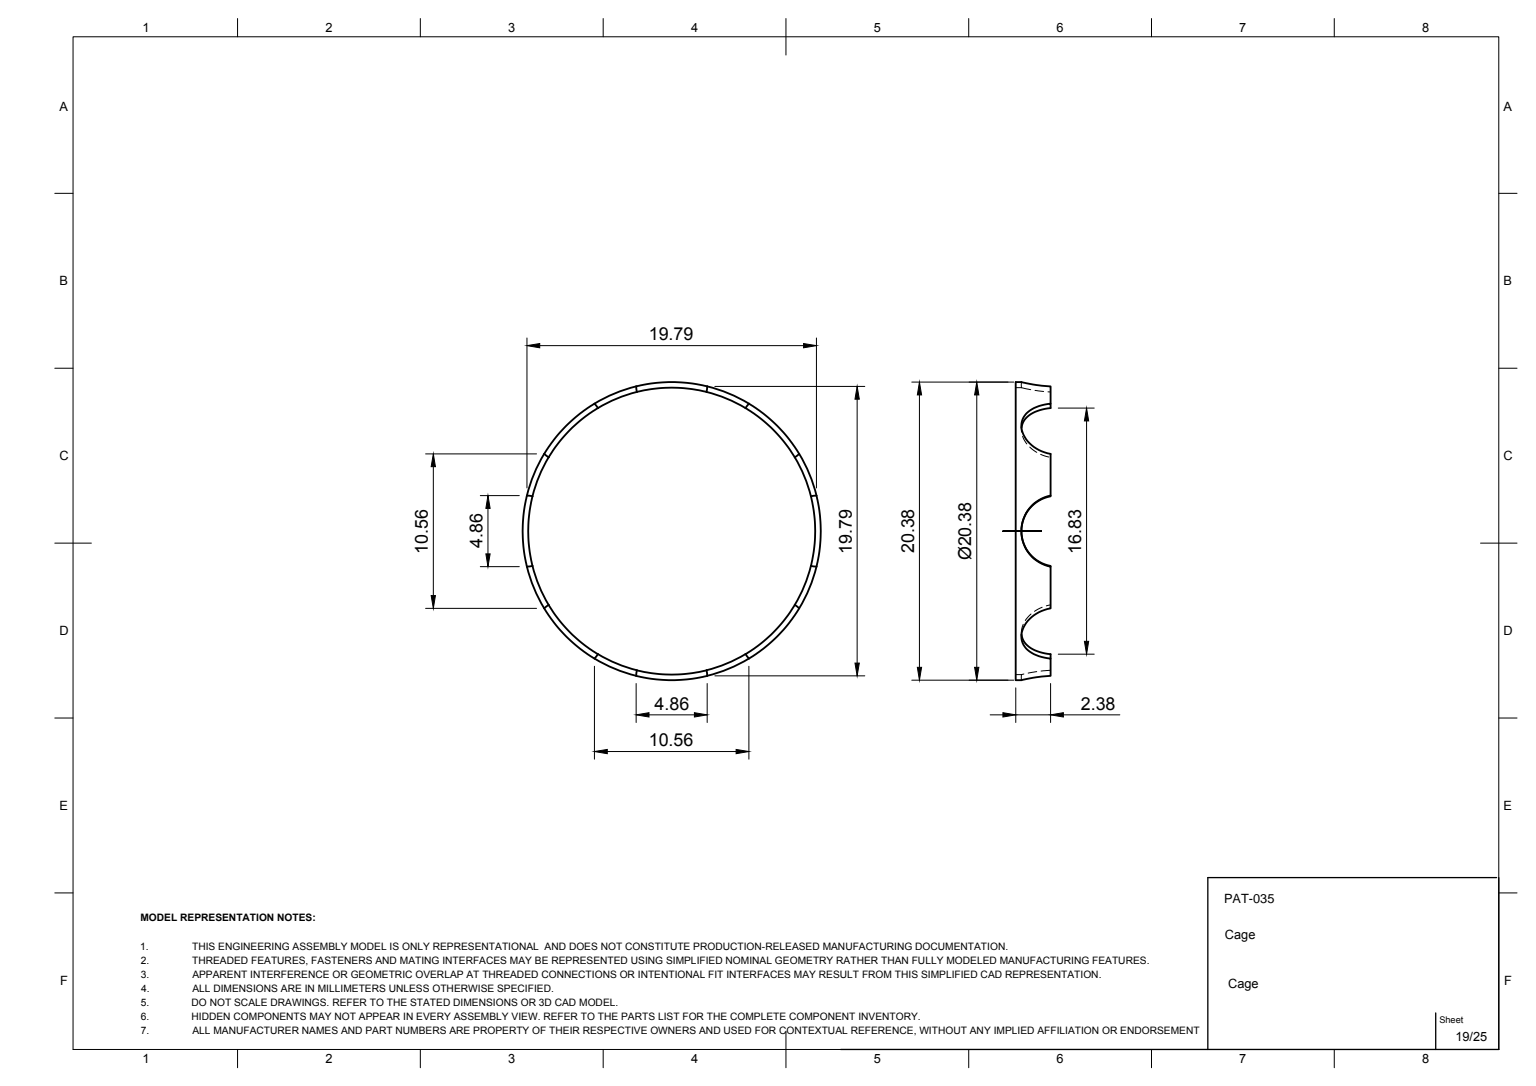
ISO-10303-21;
HEADER;
/* Generated by software containing ST-Developer
 * from STEP Tools, Inc. (www.steptools.com) 
 */

FILE_DESCRIPTION(
/* description */ ('Five-roller gravity conveyor'),
/* implementation_level */ '2;1');

FILE_NAME(
/* name */ 'Cage.step',
/* time_stamp */ '2026-10-29T15:36:43-07:00',
/* author */ (''),
/* organization */ (''),
/* preprocessor_version */ 'ST-DEVELOPER v20.2',
/* originating_system */ 'Autodesk Translation Framework v15.17.0.0',
/* authorisation */ '');

FILE_SCHEMA (('AUTOMOTIVE_DESIGN { 1 0 10303 214 3 1 1 }'));
ENDSEC;

DATA;
#10=MECHANICAL_DESIGN_GEOMETRIC_PRESENTATION_REPRESENTATION('',(#328),#7806);
#223=B_SPLINE_CURVE_WITH_KNOTS('',3,(#7017,#7018,#7019,#7020,#7021,#7022,
#7023,#7024,#7025,#7026,#7027,#7028,#7029,#7030,#7031,#7032,#7033,#7034,
#7035,#7036,#7037,#7038),.UNSPECIFIED.,.F.,.F.,(4,2,2,2,2,2,2,2,2,2,4),
(0.0473477652366656,0.126350602536658,0.189525903804987,0.252701205073317,
0.313298422430275,0.373895639787233,0.434492857144191,0.495090074501149,
0.558265375769478,0.621440677037807,0.7004435143378),.UNSPECIFIED.);
#224=B_SPLINE_CURVE_WITH_KNOTS('',3,(#7042,#7043,#7044,#7045,#7046,#7047,
#7048,#7049,#7050,#7051,#7052,#7053,#7054,#7055,#7056,#7057,#7058,#7059,
#7060,#7061,#7062,#7063),.UNSPECIFIED.,.F.,.F.,(4,2,2,2,2,2,2,2,2,2,4),
(0.0464897534940957,0.0852567806515119,0.170513561303024,0.246687263103517,
0.308657850341199,0.370628437578881,0.432599024816563,0.494569612054245,
0.570743313854739,0.656000094506251,0.694767121663666),.UNSPECIFIED.);
#225=B_SPLINE_CURVE_WITH_KNOTS('',3,(#7069,#7070,#7071,#7072,#7073,#7074,
#7075,#7076,#7077,#7078,#7079,#7080,#7081,#7082,#7083,#7084,#7085,#7086,
#7087,#7088,#7089,#7090),.UNSPECIFIED.,.F.,.F.,(4,2,2,2,2,2,2,2,2,2,4),
(0.0464897534940957,0.0852567806515118,0.170513561303024,0.246687263103517,
0.308657850341199,0.370628437578881,0.432599024816563,0.494569612054245,
0.570743313854738,0.65600009450625,0.694767121663666),.UNSPECIFIED.);
#226=B_SPLINE_CURVE_WITH_KNOTS('',3,(#7094,#7095,#7096,#7097,#7098,#7099,
#7100,#7101,#7102,#7103,#7104,#7105,#7106,#7107,#7108,#7109,#7110,#7111,
#7112,#7113,#7114,#7115),.UNSPECIFIED.,.F.,.F.,(4,2,2,2,2,2,2,2,2,2,4),
(0.0464897534940957,0.0852567806515119,0.170513561303024,0.246687263103517,
0.308657850341199,0.370628437578881,0.432599024816563,0.494569612054245,
0.570743313854739,0.656000094506251,0.694767121663666),.UNSPECIFIED.);
#227=B_SPLINE_CURVE_WITH_KNOTS('',3,(#7119,#7120,#7121,#7122,#7123,#7124,
#7125,#7126,#7127,#7128,#7129,#7130),.UNSPECIFIED.,.F.,.F.,(4,2,2,2,2,4),
(0.0464897534940957,0.0852567806515119,0.170513561303024,0.246687263103517,
0.308657850341199,0.370628437578881),.UNSPECIFIED.);
#228=B_SPLINE_CURVE_WITH_KNOTS('',3,(#7135,#7136,#7137,#7138,#7139,#7140,
#7141,#7142,#7143,#7144,#7145,#7146),.UNSPECIFIED.,.F.,.F.,(4,2,2,2,2,4),
(0.370628437578881,0.432599024816563,0.494569612054245,0.570743313854738,
0.65600009450625,0.694767121663666),.UNSPECIFIED.);
#229=B_SPLINE_CURVE_WITH_KNOTS('',3,(#7150,#7151,#7152,#7153,#7154,#7155,
#7156,#7157,#7158,#7159,#7160,#7161,#7162,#7163,#7164,#7165,#7166,#7167,
#7168,#7169,#7170,#7171),.UNSPECIFIED.,.F.,.F.,(4,2,2,2,2,2,2,2,2,2,4),
(0.0464897534940957,0.0852567806515121,0.170513561303024,0.246687263103518,
0.308657850341199,0.370628437578881,0.432599024816563,0.494569612054245,
0.570743313854738,0.65600009450625,0.694767121663666),.UNSPECIFIED.);
#230=B_SPLINE_CURVE_WITH_KNOTS('',3,(#7175,#7176,#7177,#7178,#7179,#7180,
#7181,#7182,#7183,#7184,#7185,#7186,#7187,#7188,#7189,#7190,#7191,#7192,
#7193,#7194,#7195,#7196),.UNSPECIFIED.,.F.,.F.,(4,2,2,2,2,2,2,2,2,2,4),
(0.0464897534940957,0.0852567806515119,0.170513561303024,0.246687263103517,
0.308657850341199,0.370628437578881,0.432599024816563,0.494569612054245,
0.570743313854738,0.65600009450625,0.694767121663667),.UNSPECIFIED.);
#231=B_SPLINE_CURVE_WITH_KNOTS('',3,(#7200,#7201,#7202,#7203,#7204,#7205,
#7206,#7207,#7208,#7209,#7210,#7211,#7212,#7213,#7214,#7215,#7216,#7217,
#7218,#7219,#7220,#7221),.UNSPECIFIED.,.F.,.F.,(4,2,2,2,2,2,2,2,2,2,4),
(0.0464897534940957,0.0852567806515119,0.170513561303024,0.246687263103517,
0.308657850341199,0.370628437578881,0.432599024816563,0.494569612054245,
0.570743313854738,0.65600009450625,0.694767121663666),.UNSPECIFIED.);
#232=B_SPLINE_CURVE_WITH_KNOTS('',3,(#7225,#7226,#7227,#7228,#7229,#7230,
#7231,#7232,#7233,#7234,#7235,#7236,#7237,#7238,#7239,#7240,#7241,#7242,
#7243,#7244,#7245,#7246),.UNSPECIFIED.,.F.,.F.,(4,2,2,2,2,2,2,2,2,2,4),
(0.0464897534940957,0.0852567806515119,0.170513561303024,0.246687263103517,
0.308657850341199,0.370628437578881,0.432599024816563,0.494569612054245,
0.570743313854739,0.656000094506251,0.694767121663667),.UNSPECIFIED.);
#233=B_SPLINE_CURVE_WITH_KNOTS('',3,(#7254,#7255,#7256,#7257,#7258,#7259,
#7260,#7261,#7262,#7263,#7264,#7265,#7266,#7267,#7268,#7269,#7270,#7271,
#7272,#7273,#7274,#7275),.UNSPECIFIED.,.F.,.F.,(4,2,2,2,2,2,2,2,2,2,4),
(0.0473477652366656,0.126350602536658,0.189525903804987,0.252701205073316,
0.313298422430274,0.373895639787232,0.434492857144191,0.495090074501149,
0.558265375769478,0.621440677037807,0.7004435143378),.UNSPECIFIED.);
#234=B_SPLINE_CURVE_WITH_KNOTS('',3,(#7283,#7284,#7285,#7286,#7287,#7288,
#7289,#7290,#7291,#7292,#7293,#7294,#7295,#7296,#7297,#7298,#7299,#7300,
#7301,#7302,#7303,#7304),.UNSPECIFIED.,.F.,.F.,(4,2,2,2,2,2,2,2,2,2,4),
(0.0473477652366656,0.126350602536658,0.189525903804987,0.252701205073317,
0.313298422430275,0.373895639787233,0.434492857144191,0.495090074501149,
0.558265375769478,0.621440677037807,0.7004435143378),.UNSPECIFIED.);
#235=B_SPLINE_CURVE_WITH_KNOTS('',3,(#7313,#7314,#7315,#7316,#7317,#7318,
#7319,#7320,#7321,#7322,#7323,#7324),.UNSPECIFIED.,.F.,.F.,(4,2,2,2,2,4),
(0.0473477652366656,0.126350602536658,0.189525903804987,0.252701205073316,
0.313298422430275,0.373895639787233),.UNSPECIFIED.);
#236=B_SPLINE_CURVE_WITH_KNOTS('',3,(#7326,#7327,#7328,#7329,#7330,#7331,
#7332,#7333,#7334,#7335,#7336,#7337),.UNSPECIFIED.,.F.,.F.,(4,2,2,2,2,4),
(0.373895639787233,0.434492857144191,0.495090074501149,0.558265375769478,
0.621440677037807,0.7004435143378),.UNSPECIFIED.);
#237=B_SPLINE_CURVE_WITH_KNOTS('',3,(#7344,#7345,#7346,#7347,#7348,#7349,
#7350,#7351,#7352,#7353,#7354,#7355,#7356,#7357,#7358,#7359,#7360,#7361,
#7362,#7363,#7364,#7365),.UNSPECIFIED.,.F.,.F.,(4,2,2,2,2,2,2,2,2,2,4),
(0.0473477652366656,0.126350602536658,0.189525903804987,0.252701205073316,
0.313298422430275,0.373895639787233,0.434492857144191,0.495090074501149,
0.558265375769478,0.621440677037807,0.7004435143378),.UNSPECIFIED.);
#238=B_SPLINE_CURVE_WITH_KNOTS('',3,(#7373,#7374,#7375,#7376,#7377,#7378,
#7379,#7380,#7381,#7382,#7383,#7384,#7385,#7386,#7387,#7388,#7389,#7390,
#7391,#7392,#7393,#7394),.UNSPECIFIED.,.F.,.F.,(4,2,2,2,2,2,2,2,2,2,4),
(0.0473477652366656,0.126350602536658,0.189525903804987,0.252701205073317,
0.313298422430275,0.373895639787233,0.434492857144191,0.495090074501149,
0.558265375769478,0.621440677037807,0.7004435143378),.UNSPECIFIED.);
#239=B_SPLINE_CURVE_WITH_KNOTS('',3,(#7402,#7403,#7404,#7405,#7406,#7407,
#7408,#7409,#7410,#7411,#7412,#7413,#7414,#7415,#7416,#7417,#7418,#7419,
#7420,#7421,#7422,#7423),.UNSPECIFIED.,.F.,.F.,(4,2,2,2,2,2,2,2,2,2,4),
(0.0473477652366656,0.126350602536658,0.189525903804987,0.252701205073316,
0.313298422430275,0.373895639787233,0.434492857144191,0.495090074501149,
0.558265375769478,0.621440677037807,0.7004435143378),.UNSPECIFIED.);
#240=B_SPLINE_CURVE_WITH_KNOTS('',3,(#7432,#7433,#7434,#7435,#7436,#7437,
#7438,#7439,#7440,#7441,#7442,#7443,#7444,#7445,#7446,#7447,#7448,#7449,
#7450,#7451,#7452,#7453),.UNSPECIFIED.,.F.,.F.,(4,2,2,2,2,2,2,2,2,2,4),
(0.0473477652366656,0.126350602536658,0.189525903804987,0.252701205073317,
0.313298422430275,0.373895639787233,0.434492857144191,0.495090074501149,
0.558265375769478,0.621440677037807,0.7004435143378),.UNSPECIFIED.);
#249=SPHERICAL_SURFACE('',#4677,0.247676);
#250=SPHERICAL_SURFACE('',#4693,0.247676);
#251=SPHERICAL_SURFACE('',#4698,0.247676);
#252=SPHERICAL_SURFACE('',#4703,0.247676);
#253=SPHERICAL_SURFACE('',#4708,0.247676);
#254=SPHERICAL_SURFACE('',#4713,0.247676);
#255=SPHERICAL_SURFACE('',#4718,0.247676);
#256=SPHERICAL_SURFACE('',#4726,0.247676);
#285=SHAPE_REPRESENTATION_RELATIONSHIP('SRR','None',#7923,#303);
#303=ADVANCED_BREP_SHAPE_REPRESENTATION('',(#353),#7796);
#328=STYLED_ITEM('',(#8091),#353);
#353=MANIFOLD_SOLID_BREP('Continuous crown cage',#4216);
#386=FACE_BOUND('',#1080,.T.);
#502=CIRCLE('',#4678,0.243053047864041);
#503=CIRCLE('',#4679,0.243053047864041);
#504=CIRCLE('',#4681,1.019052);
#505=CIRCLE('',#4682,1.019052);
#506=CIRCLE('',#4683,1.019052);
#507=CIRCLE('',#4684,1.019052);
#508=CIRCLE('',#4685,1.019052);
#509=CIRCLE('',#4686,1.019052);
#510=CIRCLE('',#4687,1.019052);
#511=CIRCLE('',#4688,1.019052);
#512=CIRCLE('',#4689,1.019052);
#513=CIRCLE('',#4691,0.980948);
#514=CIRCLE('',#4692,0.243053047864041);
#515=CIRCLE('',#4694,0.243053047864041);
#516=CIRCLE('',#4696,0.980948);
#517=CIRCLE('',#4697,0.243053047864041);
#518=CIRCLE('',#4699,0.243053047864041);
#519=CIRCLE('',#4701,0.980948);
#520=CIRCLE('',#4702,0.243053047864041);
#521=CIRCLE('',#4704,0.243053047864041);
#522=CIRCLE('',#4706,0.980948);
#523=CIRCLE('',#4707,0.243053047864041);
#524=CIRCLE('',#4709,0.243053047864041);
#525=CIRCLE('',#4711,0.980948);
#526=CIRCLE('',#4712,0.243053047864041);
#527=CIRCLE('',#4714,0.243053047864041);
#528=CIRCLE('',#4716,0.980948);
#529=CIRCLE('',#4717,0.243053047864041);
#530=CIRCLE('',#4719,0.243053047864041);
#531=CIRCLE('',#4721,0.980948);
#532=CIRCLE('',#4722,0.980948);
#533=CIRCLE('',#4723,0.980948);
#534=CIRCLE('',#4725,0.243053047864041);
#535=CIRCLE('',#4727,0.243053047864041);
#623=CYLINDRICAL_SURFACE('',#4680,1.019052);
#624=CYLINDRICAL_SURFACE('',#4720,0.980948);
#806=FACE_OUTER_BOUND('',#1062,.T.);
#807=FACE_OUTER_BOUND('',#1063,.T.);
#808=FACE_OUTER_BOUND('',#1064,.T.);
#809=FACE_OUTER_BOUND('',#1065,.T.);
#810=FACE_OUTER_BOUND('',#1066,.T.);
#811=FACE_OUTER_BOUND('',#1067,.T.);
#812=FACE_OUTER_BOUND('',#1068,.T.);
#813=FACE_OUTER_BOUND('',#1069,.T.);
#814=FACE_OUTER_BOUND('',#1070,.T.);
#815=FACE_OUTER_BOUND('',#1071,.T.);
#816=FACE_OUTER_BOUND('',#1072,.T.);
#817=FACE_OUTER_BOUND('',#1073,.T.);
#818=FACE_OUTER_BOUND('',#1074,.T.);
#819=FACE_OUTER_BOUND('',#1075,.T.);
#820=FACE_OUTER_BOUND('',#1076,.T.);
#821=FACE_OUTER_BOUND('',#1077,.T.);
#822=FACE_OUTER_BOUND('',#1078,.T.);
#823=FACE_OUTER_BOUND('',#1079,.T.);
#824=FACE_OUTER_BOUND('',#1081,.T.);
#1062=EDGE_LOOP('',(#3500,#3501,#3502,#3503));
#1063=EDGE_LOOP('',(#3504,#3505,#3506,#3507,#3508,#3509,#3510,#3511,#3512,
#3513,#3514,#3515,#3516,#3517,#3518,#3519,#3520,#3521,#3522,#3523));
#1064=EDGE_LOOP('',(#3524,#3525,#3526,#3527));
#1065=EDGE_LOOP('',(#3528,#3529,#3530,#3531));
#1066=EDGE_LOOP('',(#3532,#3533,#3534,#3535));
#1067=EDGE_LOOP('',(#3536,#3537,#3538,#3539));
#1068=EDGE_LOOP('',(#3540,#3541,#3542,#3543));
#1069=EDGE_LOOP('',(#3544,#3545,#3546,#3547,#3548,#3549));
#1070=EDGE_LOOP('',(#3550,#3551,#3552,#3553));
#1071=EDGE_LOOP('',(#3554,#3555,#3556,#3557));
#1072=EDGE_LOOP('',(#3558,#3559,#3560,#3561));
#1073=EDGE_LOOP('',(#3562,#3563,#3564,#3565));
#1074=EDGE_LOOP('',(#3566,#3567,#3568,#3569));
#1075=EDGE_LOOP('',(#3570,#3571,#3572,#3573));
#1076=EDGE_LOOP('',(#3574,#3575,#3576,#3577,#3578,#3579,#3580,#3581,#3582,
#3583,#3584,#3585,#3586,#3587,#3588,#3589,#3590,#3591,#3592,#3593));
#1077=EDGE_LOOP('',(#3594,#3595,#3596,#3597));
#1078=EDGE_LOOP('',(#3598,#3599,#3600,#3601));
#1079=EDGE_LOOP('',(#3602));
#1080=EDGE_LOOP('',(#3603));
#1081=EDGE_LOOP('',(#3604,#3605,#3606,#3607));
#1465=LINE('',#7132,#1806);
#1466=LINE('',#7428,#1807);
#1806=VECTOR('',#5715,1.019052);
#1807=VECTOR('',#5792,0.980948);
#2114=VERTEX_POINT('',#7015);
#2115=VERTEX_POINT('',#7016);
#2116=VERTEX_POINT('',#7039);
#2117=VERTEX_POINT('',#7041);
#2118=VERTEX_POINT('',#7066);
#2119=VERTEX_POINT('',#7068);
#2120=VERTEX_POINT('',#7091);
#2121=VERTEX_POINT('',#7093);
#2122=VERTEX_POINT('',#7116);
#2123=VERTEX_POINT('',#7118);
#2124=VERTEX_POINT('',#7131);
#2125=VERTEX_POINT('',#7134);
#2126=VERTEX_POINT('',#7147);
#2127=VERTEX_POINT('',#7149);
#2128=VERTEX_POINT('',#7172);
#2129=VERTEX_POINT('',#7174);
#2130=VERTEX_POINT('',#7197);
#2131=VERTEX_POINT('',#7199);
#2132=VERTEX_POINT('',#7222);
#2133=VERTEX_POINT('',#7224);
#2134=VERTEX_POINT('',#7249);
#2135=VERTEX_POINT('',#7253);
#2136=VERTEX_POINT('',#7278);
#2137=VERTEX_POINT('',#7282);
#2138=VERTEX_POINT('',#7307);
#2139=VERTEX_POINT('',#7311);
#2140=VERTEX_POINT('',#7312);
#2141=VERTEX_POINT('',#7339);
#2142=VERTEX_POINT('',#7343);
#2143=VERTEX_POINT('',#7368);
#2144=VERTEX_POINT('',#7372);
#2145=VERTEX_POINT('',#7397);
#2146=VERTEX_POINT('',#7401);
#2147=VERTEX_POINT('',#7426);
#2148=VERTEX_POINT('',#7429);
#2149=VERTEX_POINT('',#7431);
#2593=EDGE_CURVE('',#2114,#2115,#223,.T.);
#2594=EDGE_CURVE('',#2116,#2114,#502,.T.);
#2595=EDGE_CURVE('',#2117,#2116,#224,.T.);
#2596=EDGE_CURVE('',#2115,#2117,#503,.T.);
#2597=EDGE_CURVE('',#2118,#2116,#504,.T.);
#2598=EDGE_CURVE('',#2118,#2119,#225,.T.);
#2599=EDGE_CURVE('',#2120,#2119,#505,.T.);
#2600=EDGE_CURVE('',#2120,#2121,#226,.T.);
#2601=EDGE_CURVE('',#2122,#2121,#506,.T.);
#2602=EDGE_CURVE('',#2122,#2123,#227,.T.);
#2603=EDGE_CURVE('',#2123,#2124,#1465,.T.);
#2604=EDGE_CURVE('',#2124,#2124,#507,.T.);
#2605=EDGE_CURVE('',#2123,#2125,#228,.T.);
#2606=EDGE_CURVE('',#2126,#2125,#508,.T.);
#2607=EDGE_CURVE('',#2126,#2127,#229,.T.);
#2608=EDGE_CURVE('',#2128,#2127,#509,.T.);
#2609=EDGE_CURVE('',#2128,#2129,#230,.T.);
#2610=EDGE_CURVE('',#2130,#2129,#510,.T.);
#2611=EDGE_CURVE('',#2130,#2131,#231,.T.);
#2612=EDGE_CURVE('',#2132,#2131,#511,.T.);
#2613=EDGE_CURVE('',#2132,#2133,#232,.T.);
#2614=EDGE_CURVE('',#2117,#2133,#512,.T.);
#2615=EDGE_CURVE('',#2114,#2134,#513,.T.);
#2616=EDGE_CURVE('',#2134,#2118,#514,.T.);
#2617=EDGE_CURVE('',#2135,#2134,#233,.T.);
#2618=EDGE_CURVE('',#2119,#2135,#515,.T.);
#2619=EDGE_CURVE('',#2135,#2136,#516,.T.);
#2620=EDGE_CURVE('',#2136,#2120,#517,.T.);
#2621=EDGE_CURVE('',#2137,#2136,#234,.T.);
#2622=EDGE_CURVE('',#2121,#2137,#518,.T.);
#2623=EDGE_CURVE('',#2137,#2138,#519,.T.);
#2624=EDGE_CURVE('',#2138,#2122,#520,.T.);
#2625=EDGE_CURVE('',#2139,#2140,#235,.T.);
#2626=EDGE_CURVE('',#2125,#2139,#521,.T.);
#2627=EDGE_CURVE('',#2140,#2138,#236,.T.);
#2628=EDGE_CURVE('',#2139,#2141,#522,.T.);
#2629=EDGE_CURVE('',#2141,#2126,#523,.T.);
#2630=EDGE_CURVE('',#2142,#2141,#237,.T.);
#2631=EDGE_CURVE('',#2127,#2142,#524,.T.);
#2632=EDGE_CURVE('',#2142,#2143,#525,.T.);
#2633=EDGE_CURVE('',#2143,#2128,#526,.T.);
#2634=EDGE_CURVE('',#2144,#2143,#238,.T.);
#2635=EDGE_CURVE('',#2129,#2144,#527,.T.);
#2636=EDGE_CURVE('',#2144,#2145,#528,.T.);
#2637=EDGE_CURVE('',#2145,#2130,#529,.T.);
#2638=EDGE_CURVE('',#2146,#2145,#239,.T.);
#2639=EDGE_CURVE('',#2131,#2146,#530,.T.);
#2640=EDGE_CURVE('',#2147,#2147,#531,.T.);
#2641=EDGE_CURVE('',#2147,#2140,#1466,.T.);
#2642=EDGE_CURVE('',#2148,#2115,#532,.T.);
#2643=EDGE_CURVE('',#2148,#2149,#240,.T.);
#2644=EDGE_CURVE('',#2146,#2149,#533,.T.);
#2645=EDGE_CURVE('',#2133,#2148,#534,.T.);
#2646=EDGE_CURVE('',#2149,#2132,#535,.T.);
#3500=ORIENTED_EDGE('',*,*,#2593,.F.);
#3501=ORIENTED_EDGE('',*,*,#2594,.F.);
#3502=ORIENTED_EDGE('',*,*,#2595,.F.);
#3503=ORIENTED_EDGE('',*,*,#2596,.F.);
#3504=ORIENTED_EDGE('',*,*,#2595,.T.);
#3505=ORIENTED_EDGE('',*,*,#2597,.F.);
#3506=ORIENTED_EDGE('',*,*,#2598,.T.);
#3507=ORIENTED_EDGE('',*,*,#2599,.F.);
#3508=ORIENTED_EDGE('',*,*,#2600,.T.);
#3509=ORIENTED_EDGE('',*,*,#2601,.F.);
#3510=ORIENTED_EDGE('',*,*,#2602,.T.);
#3511=ORIENTED_EDGE('',*,*,#2603,.T.);
#3512=ORIENTED_EDGE('',*,*,#2604,.F.);
#3513=ORIENTED_EDGE('',*,*,#2603,.F.);
#3514=ORIENTED_EDGE('',*,*,#2605,.T.);
#3515=ORIENTED_EDGE('',*,*,#2606,.F.);
#3516=ORIENTED_EDGE('',*,*,#2607,.T.);
#3517=ORIENTED_EDGE('',*,*,#2608,.F.);
#3518=ORIENTED_EDGE('',*,*,#2609,.T.);
#3519=ORIENTED_EDGE('',*,*,#2610,.F.);
#3520=ORIENTED_EDGE('',*,*,#2611,.T.);
#3521=ORIENTED_EDGE('',*,*,#2612,.F.);
#3522=ORIENTED_EDGE('',*,*,#2613,.T.);
#3523=ORIENTED_EDGE('',*,*,#2614,.F.);
#3524=ORIENTED_EDGE('',*,*,#2594,.T.);
#3525=ORIENTED_EDGE('',*,*,#2615,.T.);
#3526=ORIENTED_EDGE('',*,*,#2616,.T.);
#3527=ORIENTED_EDGE('',*,*,#2597,.T.);
#3528=ORIENTED_EDGE('',*,*,#2617,.F.);
#3529=ORIENTED_EDGE('',*,*,#2618,.F.);
#3530=ORIENTED_EDGE('',*,*,#2598,.F.);
#3531=ORIENTED_EDGE('',*,*,#2616,.F.);
#3532=ORIENTED_EDGE('',*,*,#2618,.T.);
#3533=ORIENTED_EDGE('',*,*,#2619,.T.);
#3534=ORIENTED_EDGE('',*,*,#2620,.T.);
#3535=ORIENTED_EDGE('',*,*,#2599,.T.);
#3536=ORIENTED_EDGE('',*,*,#2621,.F.);
#3537=ORIENTED_EDGE('',*,*,#2622,.F.);
#3538=ORIENTED_EDGE('',*,*,#2600,.F.);
#3539=ORIENTED_EDGE('',*,*,#2620,.F.);
#3540=ORIENTED_EDGE('',*,*,#2622,.T.);
#3541=ORIENTED_EDGE('',*,*,#2623,.T.);
#3542=ORIENTED_EDGE('',*,*,#2624,.T.);
#3543=ORIENTED_EDGE('',*,*,#2601,.T.);
#3544=ORIENTED_EDGE('',*,*,#2625,.F.);
#3545=ORIENTED_EDGE('',*,*,#2626,.F.);
#3546=ORIENTED_EDGE('',*,*,#2605,.F.);
#3547=ORIENTED_EDGE('',*,*,#2602,.F.);
#3548=ORIENTED_EDGE('',*,*,#2624,.F.);
#3549=ORIENTED_EDGE('',*,*,#2627,.F.);
#3550=ORIENTED_EDGE('',*,*,#2626,.T.);
#3551=ORIENTED_EDGE('',*,*,#2628,.T.);
#3552=ORIENTED_EDGE('',*,*,#2629,.T.);
#3553=ORIENTED_EDGE('',*,*,#2606,.T.);
#3554=ORIENTED_EDGE('',*,*,#2630,.F.);
#3555=ORIENTED_EDGE('',*,*,#2631,.F.);
#3556=ORIENTED_EDGE('',*,*,#2607,.F.);
#3557=ORIENTED_EDGE('',*,*,#2629,.F.);
#3558=ORIENTED_EDGE('',*,*,#2631,.T.);
#3559=ORIENTED_EDGE('',*,*,#2632,.T.);
#3560=ORIENTED_EDGE('',*,*,#2633,.T.);
#3561=ORIENTED_EDGE('',*,*,#2608,.T.);
#3562=ORIENTED_EDGE('',*,*,#2634,.F.);
#3563=ORIENTED_EDGE('',*,*,#2635,.F.);
#3564=ORIENTED_EDGE('',*,*,#2609,.F.);
#3565=ORIENTED_EDGE('',*,*,#2633,.F.);
#3566=ORIENTED_EDGE('',*,*,#2635,.T.);
#3567=ORIENTED_EDGE('',*,*,#2636,.T.);
#3568=ORIENTED_EDGE('',*,*,#2637,.T.);
#3569=ORIENTED_EDGE('',*,*,#2610,.T.);
#3570=ORIENTED_EDGE('',*,*,#2611,.F.);
#3571=ORIENTED_EDGE('',*,*,#2637,.F.);
#3572=ORIENTED_EDGE('',*,*,#2638,.F.);
#3573=ORIENTED_EDGE('',*,*,#2639,.F.);
#3574=ORIENTED_EDGE('',*,*,#2640,.F.);
#3575=ORIENTED_EDGE('',*,*,#2641,.T.);
#3576=ORIENTED_EDGE('',*,*,#2627,.T.);
#3577=ORIENTED_EDGE('',*,*,#2623,.F.);
#3578=ORIENTED_EDGE('',*,*,#2621,.T.);
#3579=ORIENTED_EDGE('',*,*,#2619,.F.);
#3580=ORIENTED_EDGE('',*,*,#2617,.T.);
#3581=ORIENTED_EDGE('',*,*,#2615,.F.);
#3582=ORIENTED_EDGE('',*,*,#2593,.T.);
#3583=ORIENTED_EDGE('',*,*,#2642,.F.);
#3584=ORIENTED_EDGE('',*,*,#2643,.T.);
#3585=ORIENTED_EDGE('',*,*,#2644,.F.);
#3586=ORIENTED_EDGE('',*,*,#2638,.T.);
#3587=ORIENTED_EDGE('',*,*,#2636,.F.);
#3588=ORIENTED_EDGE('',*,*,#2634,.T.);
#3589=ORIENTED_EDGE('',*,*,#2632,.F.);
#3590=ORIENTED_EDGE('',*,*,#2630,.T.);
#3591=ORIENTED_EDGE('',*,*,#2628,.F.);
#3592=ORIENTED_EDGE('',*,*,#2625,.T.);
#3593=ORIENTED_EDGE('',*,*,#2641,.F.);
#3594=ORIENTED_EDGE('',*,*,#2596,.T.);
#3595=ORIENTED_EDGE('',*,*,#2614,.T.);
#3596=ORIENTED_EDGE('',*,*,#2645,.T.);
#3597=ORIENTED_EDGE('',*,*,#2642,.T.);
#3598=ORIENTED_EDGE('',*,*,#2613,.F.);
#3599=ORIENTED_EDGE('',*,*,#2646,.F.);
#3600=ORIENTED_EDGE('',*,*,#2643,.F.);
#3601=ORIENTED_EDGE('',*,*,#2645,.F.);
#3602=ORIENTED_EDGE('',*,*,#2604,.T.);
#3603=ORIENTED_EDGE('',*,*,#2640,.T.);
#3604=ORIENTED_EDGE('',*,*,#2639,.T.);
#3605=ORIENTED_EDGE('',*,*,#2644,.T.);
#3606=ORIENTED_EDGE('',*,*,#2646,.T.);
#3607=ORIENTED_EDGE('',*,*,#2612,.T.);
#3930=PLANE('',#4690);
#3931=PLANE('',#4695);
#3932=PLANE('',#4700);
#3933=PLANE('',#4705);
#3934=PLANE('',#4710);
#3935=PLANE('',#4715);
#3936=PLANE('',#4724);
#3937=PLANE('',#4728);
#3938=PLANE('',#4729);
#4121=ADVANCED_FACE('',(#806),#249,.F.);
#4122=ADVANCED_FACE('',(#807),#623,.T.);
#4123=ADVANCED_FACE('',(#808),#3930,.T.);
#4124=ADVANCED_FACE('',(#809),#250,.F.);
#4125=ADVANCED_FACE('',(#810),#3931,.T.);
#4126=ADVANCED_FACE('',(#811),#251,.F.);
#4127=ADVANCED_FACE('',(#812),#3932,.T.);
#4128=ADVANCED_FACE('',(#813),#252,.F.);
#4129=ADVANCED_FACE('',(#814),#3933,.T.);
#4130=ADVANCED_FACE('',(#815),#253,.F.);
#4131=ADVANCED_FACE('',(#816),#3934,.T.);
#4132=ADVANCED_FACE('',(#817),#254,.F.);
#4133=ADVANCED_FACE('',(#818),#3935,.T.);
#4134=ADVANCED_FACE('',(#819),#255,.F.);
#4135=ADVANCED_FACE('',(#820),#624,.F.);
#4136=ADVANCED_FACE('',(#821),#3936,.T.);
#4137=ADVANCED_FACE('',(#822),#256,.F.);
#4138=ADVANCED_FACE('',(#823,#386),#3937,.T.);
#4139=ADVANCED_FACE('',(#824),#3938,.T.);
#4216=CLOSED_SHELL('',(#4121,#4122,#4123,#4124,#4125,#4126,#4127,#4128,
#4129,#4130,#4131,#4132,#4133,#4134,#4135,#4136,#4137,#4138,#4139));
#4676=AXIS2_PLACEMENT_3D('',#7013,#5699,#5700);
#4677=AXIS2_PLACEMENT_3D('',#7014,#5701,#5702);
#4678=AXIS2_PLACEMENT_3D('',#7040,#5703,#5704);
#4679=AXIS2_PLACEMENT_3D('',#7064,#5705,#5706);
#4680=AXIS2_PLACEMENT_3D('',#7065,#5707,#5708);
#4681=AXIS2_PLACEMENT_3D('',#7067,#5709,#5710);
#4682=AXIS2_PLACEMENT_3D('',#7092,#5711,#5712);
#4683=AXIS2_PLACEMENT_3D('',#7117,#5713,#5714);
#4684=AXIS2_PLACEMENT_3D('',#7133,#5716,#5717);
#4685=AXIS2_PLACEMENT_3D('',#7148,#5718,#5719);
#4686=AXIS2_PLACEMENT_3D('',#7173,#5720,#5721);
#4687=AXIS2_PLACEMENT_3D('',#7198,#5722,#5723);
#4688=AXIS2_PLACEMENT_3D('',#7223,#5724,#5725);
#4689=AXIS2_PLACEMENT_3D('',#7247,#5726,#5727);
#4690=AXIS2_PLACEMENT_3D('',#7248,#5728,#5729);
#4691=AXIS2_PLACEMENT_3D('',#7250,#5730,#5731);
#4692=AXIS2_PLACEMENT_3D('',#7251,#5732,#5733);
#4693=AXIS2_PLACEMENT_3D('',#7252,#5734,#5735);
#4694=AXIS2_PLACEMENT_3D('',#7276,#5736,#5737);
#4695=AXIS2_PLACEMENT_3D('',#7277,#5738,#5739);
#4696=AXIS2_PLACEMENT_3D('',#7279,#5740,#5741);
#4697=AXIS2_PLACEMENT_3D('',#7280,#5742,#5743);
#4698=AXIS2_PLACEMENT_3D('',#7281,#5744,#5745);
#4699=AXIS2_PLACEMENT_3D('',#7305,#5746,#5747);
#4700=AXIS2_PLACEMENT_3D('',#7306,#5748,#5749);
#4701=AXIS2_PLACEMENT_3D('',#7308,#5750,#5751);
#4702=AXIS2_PLACEMENT_3D('',#7309,#5752,#5753);
#4703=AXIS2_PLACEMENT_3D('',#7310,#5754,#5755);
#4704=AXIS2_PLACEMENT_3D('',#7325,#5756,#5757);
#4705=AXIS2_PLACEMENT_3D('',#7338,#5758,#5759);
#4706=AXIS2_PLACEMENT_3D('',#7340,#5760,#5761);
#4707=AXIS2_PLACEMENT_3D('',#7341,#5762,#5763);
#4708=AXIS2_PLACEMENT_3D('',#7342,#5764,#5765);
#4709=AXIS2_PLACEMENT_3D('',#7366,#5766,#5767);
#4710=AXIS2_PLACEMENT_3D('',#7367,#5768,#5769);
#4711=AXIS2_PLACEMENT_3D('',#7369,#5770,#5771);
#4712=AXIS2_PLACEMENT_3D('',#7370,#5772,#5773);
#4713=AXIS2_PLACEMENT_3D('',#7371,#5774,#5775);
#4714=AXIS2_PLACEMENT_3D('',#7395,#5776,#5777);
#4715=AXIS2_PLACEMENT_3D('',#7396,#5778,#5779);
#4716=AXIS2_PLACEMENT_3D('',#7398,#5780,#5781);
#4717=AXIS2_PLACEMENT_3D('',#7399,#5782,#5783);
#4718=AXIS2_PLACEMENT_3D('',#7400,#5784,#5785);
#4719=AXIS2_PLACEMENT_3D('',#7424,#5786,#5787);
#4720=AXIS2_PLACEMENT_3D('',#7425,#5788,#5789);
#4721=AXIS2_PLACEMENT_3D('',#7427,#5790,#5791);
#4722=AXIS2_PLACEMENT_3D('',#7430,#5793,#5794);
#4723=AXIS2_PLACEMENT_3D('',#7454,#5795,#5796);
#4724=AXIS2_PLACEMENT_3D('',#7455,#5797,#5798);
#4725=AXIS2_PLACEMENT_3D('',#7456,#5799,#5800);
#4726=AXIS2_PLACEMENT_3D('',#7457,#5801,#5802);
#4727=AXIS2_PLACEMENT_3D('',#7458,#5803,#5804);
#4728=AXIS2_PLACEMENT_3D('',#7459,#5805,#5806);
#4729=AXIS2_PLACEMENT_3D('',#7460,#5807,#5808);
#5699=DIRECTION('axis',(0.,0.,1.));
#5700=DIRECTION('refdir',(1.,0.,0.));
#5701=DIRECTION('center_axis',(0.,0.,1.));
#5702=DIRECTION('ref_axis',(1.,0.,0.));
#5703=DIRECTION('center_axis',(0.,-1.,0.));
#5704=DIRECTION('ref_axis',(0.,0.,-1.));
#5705=DIRECTION('center_axis',(0.,-1.,0.));
#5706=DIRECTION('ref_axis',(0.,0.,-1.));
#5707=DIRECTION('center_axis',(0.,1.,0.));
#5708=DIRECTION('ref_axis',(1.,0.,0.));
#5709=DIRECTION('center_axis',(0.,1.,0.));
#5710=DIRECTION('ref_axis',(1.,0.,0.));
#5711=DIRECTION('center_axis',(0.,1.,0.));
#5712=DIRECTION('ref_axis',(1.,0.,0.));
#5713=DIRECTION('center_axis',(0.,1.,0.));
#5714=DIRECTION('ref_axis',(1.,0.,0.));
#5715=DIRECTION('',(0.,-1.,0.));
#5716=DIRECTION('center_axis',(0.,-1.,0.));
#5717=DIRECTION('ref_axis',(1.,0.,0.));
#5718=DIRECTION('center_axis',(0.,1.,0.));
#5719=DIRECTION('ref_axis',(1.,0.,0.));
#5720=DIRECTION('center_axis',(0.,1.,0.));
#5721=DIRECTION('ref_axis',(1.,0.,0.));
#5722=DIRECTION('center_axis',(0.,1.,0.));
#5723=DIRECTION('ref_axis',(1.,0.,0.));
#5724=DIRECTION('center_axis',(0.,1.,0.));
#5725=DIRECTION('ref_axis',(1.,0.,0.));
#5726=DIRECTION('center_axis',(0.,1.,0.));
#5727=DIRECTION('ref_axis',(1.,0.,0.));
#5728=DIRECTION('center_axis',(0.,1.,0.));
#5729=DIRECTION('ref_axis',(1.,0.,0.));
#5730=DIRECTION('center_axis',(0.,-1.,0.));
#5731=DIRECTION('ref_axis',(1.,0.,0.));
#5732=DIRECTION('center_axis',(0.,-1.,0.));
#5733=DIRECTION('ref_axis',(0.,0.,-1.));
#5734=DIRECTION('center_axis',(6.12323399573677E-17,0.,1.));
#5735=DIRECTION('ref_axis',(1.,0.,0.));
#5736=DIRECTION('center_axis',(0.,-1.,0.));
#5737=DIRECTION('ref_axis',(0.,0.,-1.));
#5738=DIRECTION('center_axis',(0.,1.,0.));
#5739=DIRECTION('ref_axis',(1.,0.,0.));
#5740=DIRECTION('center_axis',(0.,-1.,0.));
#5741=DIRECTION('ref_axis',(1.,0.,0.));
#5742=DIRECTION('center_axis',(0.,-1.,0.));
#5743=DIRECTION('ref_axis',(0.,0.,-1.));
#5744=DIRECTION('center_axis',(0.,0.,1.));
#5745=DIRECTION('ref_axis',(1.,0.,0.));
#5746=DIRECTION('center_axis',(0.,-1.,0.));
#5747=DIRECTION('ref_axis',(0.,0.,-1.));
#5748=DIRECTION('center_axis',(0.,1.,0.));
#5749=DIRECTION('ref_axis',(1.,0.,0.));
#5750=DIRECTION('center_axis',(0.,-1.,0.));
#5751=DIRECTION('ref_axis',(1.,0.,0.));
#5752=DIRECTION('center_axis',(0.,-1.,0.));
#5753=DIRECTION('ref_axis',(0.,0.,-1.));
#5754=DIRECTION('center_axis',(0.,0.,1.));
#5755=DIRECTION('ref_axis',(1.,0.,0.));
#5756=DIRECTION('center_axis',(0.,-1.,0.));
#5757=DIRECTION('ref_axis',(0.,0.,-1.));
#5758=DIRECTION('center_axis',(0.,1.,0.));
#5759=DIRECTION('ref_axis',(1.,0.,0.));
#5760=DIRECTION('center_axis',(0.,-1.,0.));
#5761=DIRECTION('ref_axis',(1.,0.,0.));
#5762=DIRECTION('center_axis',(0.,-1.,0.));
#5763=DIRECTION('ref_axis',(0.,0.,-1.));
#5764=DIRECTION('center_axis',(0.,0.,1.));
#5765=DIRECTION('ref_axis',(1.,0.,0.));
#5766=DIRECTION('center_axis',(0.,-1.,0.));
#5767=DIRECTION('ref_axis',(0.,0.,-1.));
#5768=DIRECTION('center_axis',(0.,1.,0.));
#5769=DIRECTION('ref_axis',(1.,0.,0.));
#5770=DIRECTION('center_axis',(0.,-1.,0.));
#5771=DIRECTION('ref_axis',(1.,0.,0.));
#5772=DIRECTION('center_axis',(0.,-1.,0.));
#5773=DIRECTION('ref_axis',(0.,0.,-1.));
#5774=DIRECTION('center_axis',(6.12323399573676E-17,0.,1.));
#5775=DIRECTION('ref_axis',(1.,0.,0.));
#5776=DIRECTION('center_axis',(0.,-1.,0.));
#5777=DIRECTION('ref_axis',(0.,0.,-1.));
#5778=DIRECTION('center_axis',(0.,1.,0.));
#5779=DIRECTION('ref_axis',(1.,0.,0.));
#5780=DIRECTION('center_axis',(0.,-1.,0.));
#5781=DIRECTION('ref_axis',(1.,0.,0.));
#5782=DIRECTION('center_axis',(0.,-1.,0.));
#5783=DIRECTION('ref_axis',(0.,0.,-1.));
#5784=DIRECTION('center_axis',(0.,0.,1.));
#5785=DIRECTION('ref_axis',(1.,0.,0.));
#5786=DIRECTION('center_axis',(0.,-1.,0.));
#5787=DIRECTION('ref_axis',(0.,0.,-1.));
#5788=DIRECTION('center_axis',(0.,1.,0.));
#5789=DIRECTION('ref_axis',(1.,0.,0.));
#5790=DIRECTION('center_axis',(0.,1.,0.));
#5791=DIRECTION('ref_axis',(1.,0.,0.));
#5792=DIRECTION('',(0.,1.,0.));
#5793=DIRECTION('center_axis',(0.,-1.,0.));
#5794=DIRECTION('ref_axis',(1.,0.,0.));
#5795=DIRECTION('center_axis',(0.,-1.,0.));
#5796=DIRECTION('ref_axis',(1.,0.,0.));
#5797=DIRECTION('center_axis',(0.,1.,0.));
#5798=DIRECTION('ref_axis',(1.,0.,0.));
#5799=DIRECTION('center_axis',(0.,-1.,0.));
#5800=DIRECTION('ref_axis',(0.,0.,-1.));
#5801=DIRECTION('center_axis',(0.,0.,1.));
#5802=DIRECTION('ref_axis',(1.,0.,0.));
#5803=DIRECTION('center_axis',(0.,-1.,0.));
#5804=DIRECTION('ref_axis',(0.,0.,-1.));
#5805=DIRECTION('center_axis',(0.,-1.,0.));
#5806=DIRECTION('ref_axis',(-1.,0.,0.));
#5807=DIRECTION('center_axis',(0.,1.,0.));
#5808=DIRECTION('ref_axis',(1.,0.,0.));
#7013=CARTESIAN_POINT('',(0.,0.,0.));
#7014=CARTESIAN_POINT('Origin',(0.707106781186547,0.,0.707106781186548));
#7015=CARTESIAN_POINT('',(0.504455939115715,-0.04763,0.841298510752802));
#7016=CARTESIAN_POINT('',(0.841298510752802,-0.04763,0.504455939115715));
#7017=CARTESIAN_POINT('Ctrl Pts',(0.504455939115715,-0.04763,0.841298510752802));
#7018=CARTESIAN_POINT('Ctrl Pts',(0.508899795931835,-0.0740444353928835,
0.838633903678357));
#7019=CARTESIAN_POINT('Ctrl Pts',(0.517157748491652,-0.0999305678883309,
0.833661031856294));
#7020=CARTESIAN_POINT('Ctrl Pts',(0.537715343527944,-0.142345102874864,
0.820511285096538));
#7021=CARTESIAN_POINT('Ctrl Pts',(0.548874290046456,-0.159766064500479,
0.813159949759));
#7022=CARTESIAN_POINT('Ctrl Pts',(0.573915184558107,-0.190326085855194,
0.795684265985089));
#7023=CARTESIAN_POINT('Ctrl Pts',(0.587792702767295,-0.203463743702801,
0.78555112003688));
#7024=CARTESIAN_POINT('Ctrl Pts',(0.615966552324775,-0.224161999508995,
0.763642258217233));
#7025=CARTESIAN_POINT('Ctrl Pts',(0.631684198665438,-0.232861760990032,
0.750785745543687));
#7026=CARTESIAN_POINT('Ctrl Pts',(0.663382628119203,-0.244251601209411,
0.722929908501543));
#7027=CARTESIAN_POINT('Ctrl Pts',(0.679352081686668,-0.246942143572133,
0.707917883896095));
#7028=CARTESIAN_POINT('Ctrl Pts',(0.707917883896095,-0.246942143572133,
0.679352081686668));
#7029=CARTESIAN_POINT('Ctrl Pts',(0.722929908501543,-0.244251601209411,
0.663382628119203));
#7030=CARTESIAN_POINT('Ctrl Pts',(0.750785745543687,-0.232861760990032,
0.631684198665439));
#7031=CARTESIAN_POINT('Ctrl Pts',(0.763642258217232,-0.224161999508995,
0.615966552324775));
#7032=CARTESIAN_POINT('Ctrl Pts',(0.78555112003688,-0.203463743702801,0.587792702767295));
#7033=CARTESIAN_POINT('Ctrl Pts',(0.795684265985088,-0.190326085855194,
0.573915184558108));
#7034=CARTESIAN_POINT('Ctrl Pts',(0.813159949759,-0.15976606450048,0.548874290046456));
#7035=CARTESIAN_POINT('Ctrl Pts',(0.820511285096538,-0.142345102874864,
0.537715343527944));
#7036=CARTESIAN_POINT('Ctrl Pts',(0.833661031856294,-0.099930567888331,
0.517157748491653));
#7037=CARTESIAN_POINT('Ctrl Pts',(0.838633903678357,-0.0740444353928835,
0.508899795931835));
#7038=CARTESIAN_POINT('Ctrl Pts',(0.841298510752801,-0.0476299999999999,
0.504455939115715));
#7039=CARTESIAN_POINT('',(0.528110872004958,-0.04763,0.871530771444223));
#7040=CARTESIAN_POINT('Origin',(0.707106781186547,-0.04763,0.707106781186548));
#7041=CARTESIAN_POINT('',(0.871530771444223,-0.04763,0.528110872004959));
#7042=CARTESIAN_POINT('Ctrl Pts',(0.871530771444223,-0.0476300000000001,
0.528110872004958));
#7043=CARTESIAN_POINT('Ctrl Pts',(0.87014664509073,-0.0609922781173483,
0.530395067942936));
#7044=CARTESIAN_POINT('Ctrl Pts',(0.868149331745851,-0.0742967091364493,
0.533674141594226));
#7045=CARTESIAN_POINT('Ctrl Pts',(0.85981294420286,-0.115492077056649,0.54708917182331));
#7046=CARTESIAN_POINT('Ctrl Pts',(0.850993704737257,-0.141695629206859,
0.560922177770136));
#7047=CARTESIAN_POINT('Ctrl Pts',(0.830754510485543,-0.181890537957859,
0.590422647829571));
#7048=CARTESIAN_POINT('Ctrl Pts',(0.816896541396381,-0.201072148666545,
0.609616703125488));
#7049=CARTESIAN_POINT('Ctrl Pts',(0.792310597819928,-0.223955109275652,
0.641117951819998));
#7050=CARTESIAN_POINT('Ctrl Pts',(0.779109323683612,-0.232742381310829,
0.657208095763053));
#7051=CARTESIAN_POINT('Ctrl Pts',(0.750552691816206,-0.244234834628584,
0.68964083160521));
#7052=CARTESIAN_POINT('Ctrl Pts',(0.735185187071673,-0.246942143572133,
0.705971972091755));
#7053=CARTESIAN_POINT('Ctrl Pts',(0.705971972091754,-0.246942143572133,
0.735185187071673));
#7054=CARTESIAN_POINT('Ctrl Pts',(0.689640831605209,-0.244234834628584,
0.750552691816206));
#7055=CARTESIAN_POINT('Ctrl Pts',(0.657208095763052,-0.232742381310829,
0.779109323683612));
#7056=CARTESIAN_POINT('Ctrl Pts',(0.641117951819998,-0.223955109275652,
0.792310597819928));
#7057=CARTESIAN_POINT('Ctrl Pts',(0.609616703125487,-0.201072148666545,
0.816896541396382));
#7058=CARTESIAN_POINT('Ctrl Pts',(0.590422647829571,-0.181890537957858,
0.830754510485544));
#7059=CARTESIAN_POINT('Ctrl Pts',(0.560922177770135,-0.141695629206858,
0.850993704737257));
#7060=CARTESIAN_POINT('Ctrl Pts',(0.547089171823309,-0.115492077056649,
0.859812944202861));
#7061=CARTESIAN_POINT('Ctrl Pts',(0.533674141594226,-0.0742967091364491,
0.868149331745852));
#7062=CARTESIAN_POINT('Ctrl Pts',(0.530395067942936,-0.0609922781173483,
0.870146645090731));
#7063=CARTESIAN_POINT('Ctrl Pts',(0.528110872004958,-0.0476300000000001,
0.871530771444223));
#7064=CARTESIAN_POINT('Origin',(0.707106781186547,-0.04763,0.707106781186548));
#7065=CARTESIAN_POINT('Origin',(0.,-0.166705,0.));
#7066=CARTESIAN_POINT('',(0.242834539687906,-0.04763,0.989696097314));
#7067=CARTESIAN_POINT('Origin',(0.,-0.04763,0.));
#7068=CARTESIAN_POINT('',(-0.242834539687907,-0.04763,0.989696097314));
#7069=CARTESIAN_POINT('Ctrl Pts',(0.242834539687906,-0.04763,0.989696097314));
#7070=CARTESIAN_POINT('Ctrl Pts',(0.24024064412003,-0.0609922781173483,
0.990332542620729));
#7071=CARTESIAN_POINT('Ctrl Pts',(0.236509675094874,-0.0742967091364492,
0.991238884025248));
#7072=CARTESIAN_POINT('Ctrl Pts',(0.221129100087819,-0.115492077056649,
0.994830026707808));
#7073=CARTESIAN_POINT('Ctrl Pts',(0.205111543747588,-0.141695629206859,
0.998375294985966));
#7074=CARTESIAN_POINT('Ctrl Pts',(0.169940289819232,-0.181890537957859,
1.00492400591205));
#7075=CARTESIAN_POINT('Ctrl Pts',(0.1465689792446,-0.201072148666545,1.00869718865384));
#7076=CARTESIAN_POINT('Ctrl Pts',(0.106909345252087,-0.223955109275652,
1.01358704779679));
#7077=CARTESIAN_POINT('Ctrl Pts',(0.0861971848975941,-0.232742381310829,
1.0156297872271));
#7078=CARTESIAN_POINT('Ctrl Pts',(0.0430711894098822,-0.244234834628584,
1.01837060663223));
#7079=CARTESIAN_POINT('Ctrl Pts',(0.0206568624125605,-0.246942143572133,
1.019052));
#7080=CARTESIAN_POINT('Ctrl Pts',(-0.0206568624125608,-0.246942143572133,
1.019052));
#7081=CARTESIAN_POINT('Ctrl Pts',(-0.0430711894098825,-0.244234834628584,
1.01837060663223));
#7082=CARTESIAN_POINT('Ctrl Pts',(-0.0861971848975943,-0.232742381310829,
1.0156297872271));
#7083=CARTESIAN_POINT('Ctrl Pts',(-0.106909345252088,-0.223955109275652,
1.01358704779679));
#7084=CARTESIAN_POINT('Ctrl Pts',(-0.1465689792446,-0.201072148666545,1.00869718865384));
#7085=CARTESIAN_POINT('Ctrl Pts',(-0.169940289819232,-0.181890537957859,
1.00492400591205));
#7086=CARTESIAN_POINT('Ctrl Pts',(-0.205111543747588,-0.141695629206859,
0.998375294985966));
#7087=CARTESIAN_POINT('Ctrl Pts',(-0.221129100087819,-0.115492077056649,
0.994830026707808));
#7088=CARTESIAN_POINT('Ctrl Pts',(-0.236509675094875,-0.0742967091364493,
0.991238884025248));
#7089=CARTESIAN_POINT('Ctrl Pts',(-0.24024064412003,-0.0609922781173483,
0.990332542620729));
#7090=CARTESIAN_POINT('Ctrl Pts',(-0.242834539687907,-0.04763,0.989696097314));
#7091=CARTESIAN_POINT('',(-0.528110872004959,-0.04763,0.871530771444223));
#7092=CARTESIAN_POINT('Origin',(0.,-0.04763,0.));
#7093=CARTESIAN_POINT('',(-0.871530771444223,-0.04763,0.528110872004958));
#7094=CARTESIAN_POINT('Ctrl Pts',(-0.528110872004958,-0.0476300000000001,
0.871530771444223));
#7095=CARTESIAN_POINT('Ctrl Pts',(-0.530395067942936,-0.0609922781173484,
0.87014664509073));
#7096=CARTESIAN_POINT('Ctrl Pts',(-0.533674141594226,-0.0742967091364493,
0.868149331745851));
#7097=CARTESIAN_POINT('Ctrl Pts',(-0.54708917182331,-0.115492077056649,
0.85981294420286));
#7098=CARTESIAN_POINT('Ctrl Pts',(-0.560922177770136,-0.141695629206859,
0.850993704737257));
#7099=CARTESIAN_POINT('Ctrl Pts',(-0.590422647829571,-0.181890537957859,
0.830754510485543));
#7100=CARTESIAN_POINT('Ctrl Pts',(-0.609616703125488,-0.201072148666545,
0.816896541396381));
#7101=CARTESIAN_POINT('Ctrl Pts',(-0.641117951819998,-0.223955109275652,
0.792310597819928));
#7102=CARTESIAN_POINT('Ctrl Pts',(-0.657208095763053,-0.232742381310829,
0.779109323683611));
#7103=CARTESIAN_POINT('Ctrl Pts',(-0.68964083160521,-0.244234834628584,
0.750552691816205));
#7104=CARTESIAN_POINT('Ctrl Pts',(-0.705971972091755,-0.246942143572133,
0.735185187071673));
#7105=CARTESIAN_POINT('Ctrl Pts',(-0.735185187071673,-0.246942143572133,
0.705971972091754));
#7106=CARTESIAN_POINT('Ctrl Pts',(-0.750552691816206,-0.244234834628584,
0.689640831605209));
#7107=CARTESIAN_POINT('Ctrl Pts',(-0.779109323683612,-0.232742381310829,
0.657208095763052));
#7108=CARTESIAN_POINT('Ctrl Pts',(-0.792310597819928,-0.223955109275652,
0.641117951819998));
#7109=CARTESIAN_POINT('Ctrl Pts',(-0.816896541396382,-0.201072148666545,
0.609616703125487));
#7110=CARTESIAN_POINT('Ctrl Pts',(-0.830754510485544,-0.181890537957858,
0.590422647829571));
#7111=CARTESIAN_POINT('Ctrl Pts',(-0.850993704737257,-0.141695629206858,
0.560922177770135));
#7112=CARTESIAN_POINT('Ctrl Pts',(-0.859812944202861,-0.115492077056649,
0.547089171823309));
#7113=CARTESIAN_POINT('Ctrl Pts',(-0.868149331745852,-0.0742967091364491,
0.533674141594226));
#7114=CARTESIAN_POINT('Ctrl Pts',(-0.870146645090731,-0.0609922781173483,
0.530395067942936));
#7115=CARTESIAN_POINT('Ctrl Pts',(-0.871530771444223,-0.04763,0.528110872004958));
#7116=CARTESIAN_POINT('',(-0.989696097314,-0.04763,0.242834539687906));
#7117=CARTESIAN_POINT('Origin',(0.,-0.04763,0.));
#7118=CARTESIAN_POINT('',(-1.019052,-0.246942143572133,1.248489836334E-16));
#7119=CARTESIAN_POINT('Ctrl Pts',(-0.989696097314,-0.04763,0.242834539687906));
#7120=CARTESIAN_POINT('Ctrl Pts',(-0.990332542620729,-0.0609922781173483,
0.24024064412003));
#7121=CARTESIAN_POINT('Ctrl Pts',(-0.991238884025248,-0.0742967091364492,
0.236509675094874));
#7122=CARTESIAN_POINT('Ctrl Pts',(-0.994830026707808,-0.115492077056649,
0.221129100087819));
#7123=CARTESIAN_POINT('Ctrl Pts',(-0.998375294985966,-0.141695629206859,
0.205111543747588));
#7124=CARTESIAN_POINT('Ctrl Pts',(-1.00492400591205,-0.181890537957859,
0.169940289819232));
#7125=CARTESIAN_POINT('Ctrl Pts',(-1.00869718865384,-0.201072148666545,
0.1465689792446));
#7126=CARTESIAN_POINT('Ctrl Pts',(-1.01358704779679,-0.223955109275652,
0.106909345252088));
#7127=CARTESIAN_POINT('Ctrl Pts',(-1.0156297872271,-0.232742381310829,0.0861971848975944));
#7128=CARTESIAN_POINT('Ctrl Pts',(-1.01837060663223,-0.244234834628584,
0.0430711894098825));
#7129=CARTESIAN_POINT('Ctrl Pts',(-1.019052,-0.246942143572133,0.0206568624125608));
#7130=CARTESIAN_POINT('Ctrl Pts',(-1.019052,-0.246942143572133,1.2490009027033E-16));
#7131=CARTESIAN_POINT('',(-1.019052,-0.28578,1.24797876996471E-16));
#7132=CARTESIAN_POINT('',(-1.019052,-0.166705,1.24797876996471E-16));
#7133=CARTESIAN_POINT('Origin',(0.,-0.28578,0.));
#7134=CARTESIAN_POINT('',(-0.989696097314,-0.04763,-0.242834539687906));
#7135=CARTESIAN_POINT('Ctrl Pts',(-1.019052,-0.246942143572133,1.2490009027033E-16));
#7136=CARTESIAN_POINT('Ctrl Pts',(-1.019052,-0.246942143572133,-0.0206568624125605));
#7137=CARTESIAN_POINT('Ctrl Pts',(-1.01837060663223,-0.244234834628584,
-0.0430711894098822));
#7138=CARTESIAN_POINT('Ctrl Pts',(-1.0156297872271,-0.232742381310829,-0.0861971848975941));
#7139=CARTESIAN_POINT('Ctrl Pts',(-1.01358704779679,-0.223955109275652,
-0.106909345252087));
#7140=CARTESIAN_POINT('Ctrl Pts',(-1.00869718865384,-0.201072148666546,
-0.1465689792446));
#7141=CARTESIAN_POINT('Ctrl Pts',(-1.00492400591205,-0.181890537957859,
-0.169940289819232));
#7142=CARTESIAN_POINT('Ctrl Pts',(-0.998375294985966,-0.141695629206859,
-0.205111543747588));
#7143=CARTESIAN_POINT('Ctrl Pts',(-0.994830026707808,-0.11549207705665,
-0.221129100087819));
#7144=CARTESIAN_POINT('Ctrl Pts',(-0.991238884025248,-0.0742967091364495,
-0.236509675094874));
#7145=CARTESIAN_POINT('Ctrl Pts',(-0.990332542620729,-0.0609922781173484,
-0.24024064412003));
#7146=CARTESIAN_POINT('Ctrl Pts',(-0.989696097314,-0.0476300000000001,-0.242834539687907));
#7147=CARTESIAN_POINT('',(-0.871530771444223,-0.04763,-0.528110872004958));
#7148=CARTESIAN_POINT('Origin',(0.,-0.04763,0.));
#7149=CARTESIAN_POINT('',(-0.528110872004958,-0.04763,-0.871530771444223));
#7150=CARTESIAN_POINT('Ctrl Pts',(-0.871530771444223,-0.0476300000000001,
-0.528110872004958));
#7151=CARTESIAN_POINT('Ctrl Pts',(-0.87014664509073,-0.0609922781173484,
-0.530395067942936));
#7152=CARTESIAN_POINT('Ctrl Pts',(-0.868149331745851,-0.0742967091364494,
-0.533674141594226));
#7153=CARTESIAN_POINT('Ctrl Pts',(-0.85981294420286,-0.115492077056649,
-0.54708917182331));
#7154=CARTESIAN_POINT('Ctrl Pts',(-0.850993704737257,-0.141695629206859,
-0.560922177770136));
#7155=CARTESIAN_POINT('Ctrl Pts',(-0.830754510485543,-0.181890537957859,
-0.590422647829571));
#7156=CARTESIAN_POINT('Ctrl Pts',(-0.816896541396381,-0.201072148666546,
-0.609616703125488));
#7157=CARTESIAN_POINT('Ctrl Pts',(-0.792310597819928,-0.223955109275652,
-0.641117951819999));
#7158=CARTESIAN_POINT('Ctrl Pts',(-0.779109323683611,-0.232742381310829,
-0.657208095763053));
#7159=CARTESIAN_POINT('Ctrl Pts',(-0.750552691816205,-0.244234834628584,
-0.68964083160521));
#7160=CARTESIAN_POINT('Ctrl Pts',(-0.735185187071673,-0.246942143572133,
-0.705971972091755));
#7161=CARTESIAN_POINT('Ctrl Pts',(-0.705971972091754,-0.246942143572133,
-0.735185187071673));
#7162=CARTESIAN_POINT('Ctrl Pts',(-0.68964083160521,-0.244234834628584,
-0.750552691816206));
#7163=CARTESIAN_POINT('Ctrl Pts',(-0.657208095763052,-0.232742381310829,
-0.779109323683612));
#7164=CARTESIAN_POINT('Ctrl Pts',(-0.641117951819998,-0.223955109275652,
-0.792310597819928));
#7165=CARTESIAN_POINT('Ctrl Pts',(-0.609616703125488,-0.201072148666545,
-0.816896541396381));
#7166=CARTESIAN_POINT('Ctrl Pts',(-0.590422647829571,-0.181890537957859,
-0.830754510485543));
#7167=CARTESIAN_POINT('Ctrl Pts',(-0.560922177770136,-0.141695629206859,
-0.850993704737257));
#7168=CARTESIAN_POINT('Ctrl Pts',(-0.54708917182331,-0.115492077056649,
-0.85981294420286));
#7169=CARTESIAN_POINT('Ctrl Pts',(-0.533674141594226,-0.0742967091364494,
-0.868149331745852));
#7170=CARTESIAN_POINT('Ctrl Pts',(-0.530395067942936,-0.0609922781173484,
-0.870146645090731));
#7171=CARTESIAN_POINT('Ctrl Pts',(-0.528110872004958,-0.0476300000000001,
-0.871530771444223));
#7172=CARTESIAN_POINT('',(-0.242834539687906,-0.04763,-0.989696097314));
#7173=CARTESIAN_POINT('Origin',(0.,-0.04763,0.));
#7174=CARTESIAN_POINT('',(0.242834539687906,-0.04763,-0.989696097314));
#7175=CARTESIAN_POINT('Ctrl Pts',(-0.242834539687907,-0.04763,-0.989696097314));
#7176=CARTESIAN_POINT('Ctrl Pts',(-0.24024064412003,-0.0609922781173483,
-0.990332542620729));
#7177=CARTESIAN_POINT('Ctrl Pts',(-0.236509675094874,-0.0742967091364493,
-0.991238884025248));
#7178=CARTESIAN_POINT('Ctrl Pts',(-0.221129100087819,-0.115492077056649,
-0.994830026707808));
#7179=CARTESIAN_POINT('Ctrl Pts',(-0.205111543747588,-0.141695629206859,
-0.998375294985966));
#7180=CARTESIAN_POINT('Ctrl Pts',(-0.169940289819232,-0.181890537957859,
-1.00492400591205));
#7181=CARTESIAN_POINT('Ctrl Pts',(-0.1465689792446,-0.201072148666545,-1.00869718865384));
#7182=CARTESIAN_POINT('Ctrl Pts',(-0.106909345252087,-0.223955109275652,
-1.01358704779679));
#7183=CARTESIAN_POINT('Ctrl Pts',(-0.0861971848975942,-0.232742381310829,
-1.0156297872271));
#7184=CARTESIAN_POINT('Ctrl Pts',(-0.0430711894098823,-0.244234834628584,
-1.01837060663223));
#7185=CARTESIAN_POINT('Ctrl Pts',(-0.0206568624125606,-0.246942143572133,
-1.019052));
#7186=CARTESIAN_POINT('Ctrl Pts',(0.0206568624125607,-0.246942143572133,
-1.019052));
#7187=CARTESIAN_POINT('Ctrl Pts',(0.0430711894098824,-0.244234834628584,
-1.01837060663223));
#7188=CARTESIAN_POINT('Ctrl Pts',(0.0861971848975943,-0.232742381310829,
-1.0156297872271));
#7189=CARTESIAN_POINT('Ctrl Pts',(0.106909345252088,-0.223955109275652,
-1.01358704779679));
#7190=CARTESIAN_POINT('Ctrl Pts',(0.1465689792446,-0.201072148666545,-1.00869718865384));
#7191=CARTESIAN_POINT('Ctrl Pts',(0.169940289819232,-0.181890537957859,
-1.00492400591205));
#7192=CARTESIAN_POINT('Ctrl Pts',(0.205111543747588,-0.141695629206859,
-0.998375294985966));
#7193=CARTESIAN_POINT('Ctrl Pts',(0.221129100087819,-0.115492077056649,
-0.994830026707808));
#7194=CARTESIAN_POINT('Ctrl Pts',(0.236509675094874,-0.0742967091364493,
-0.991238884025248));
#7195=CARTESIAN_POINT('Ctrl Pts',(0.24024064412003,-0.0609922781173484,
-0.990332542620729));
#7196=CARTESIAN_POINT('Ctrl Pts',(0.242834539687907,-0.04763,-0.989696097314));
#7197=CARTESIAN_POINT('',(0.528110872004958,-0.04763,-0.871530771444223));
#7198=CARTESIAN_POINT('Origin',(0.,-0.04763,0.));
#7199=CARTESIAN_POINT('',(0.871530771444223,-0.04763,-0.528110872004958));
#7200=CARTESIAN_POINT('Ctrl Pts',(0.528110872004958,-0.0476300000000001,
-0.871530771444223));
#7201=CARTESIAN_POINT('Ctrl Pts',(0.530395067942936,-0.0609922781173484,
-0.870146645090731));
#7202=CARTESIAN_POINT('Ctrl Pts',(0.533674141594226,-0.0742967091364493,
-0.868149331745851));
#7203=CARTESIAN_POINT('Ctrl Pts',(0.54708917182331,-0.115492077056649,-0.85981294420286));
#7204=CARTESIAN_POINT('Ctrl Pts',(0.560922177770136,-0.141695629206859,
-0.850993704737257));
#7205=CARTESIAN_POINT('Ctrl Pts',(0.590422647829571,-0.181890537957859,
-0.830754510485543));
#7206=CARTESIAN_POINT('Ctrl Pts',(0.609616703125488,-0.201072148666545,
-0.816896541396381));
#7207=CARTESIAN_POINT('Ctrl Pts',(0.641117951819998,-0.223955109275652,
-0.792310597819928));
#7208=CARTESIAN_POINT('Ctrl Pts',(0.657208095763053,-0.232742381310829,
-0.779109323683612));
#7209=CARTESIAN_POINT('Ctrl Pts',(0.68964083160521,-0.244234834628584,-0.750552691816206));
#7210=CARTESIAN_POINT('Ctrl Pts',(0.705971972091755,-0.246942143572133,
-0.735185187071673));
#7211=CARTESIAN_POINT('Ctrl Pts',(0.735185187071673,-0.246942143572133,
-0.705971972091754));
#7212=CARTESIAN_POINT('Ctrl Pts',(0.750552691816206,-0.244234834628584,
-0.68964083160521));
#7213=CARTESIAN_POINT('Ctrl Pts',(0.779109323683612,-0.232742381310829,
-0.657208095763053));
#7214=CARTESIAN_POINT('Ctrl Pts',(0.792310597819928,-0.223955109275652,
-0.641117951819998));
#7215=CARTESIAN_POINT('Ctrl Pts',(0.816896541396381,-0.201072148666545,
-0.609616703125488));
#7216=CARTESIAN_POINT('Ctrl Pts',(0.830754510485543,-0.181890537957859,
-0.590422647829571));
#7217=CARTESIAN_POINT('Ctrl Pts',(0.850993704737257,-0.141695629206859,
-0.560922177770136));
#7218=CARTESIAN_POINT('Ctrl Pts',(0.85981294420286,-0.115492077056649,-0.54708917182331));
#7219=CARTESIAN_POINT('Ctrl Pts',(0.868149331745851,-0.0742967091364493,
-0.533674141594226));
#7220=CARTESIAN_POINT('Ctrl Pts',(0.870146645090731,-0.0609922781173484,
-0.530395067942936));
#7221=CARTESIAN_POINT('Ctrl Pts',(0.871530771444223,-0.0476300000000001,
-0.528110872004958));
#7222=CARTESIAN_POINT('',(0.989696097314,-0.04763,-0.242834539687906));
#7223=CARTESIAN_POINT('Origin',(0.,-0.04763,0.));
#7224=CARTESIAN_POINT('',(0.989696097314,-0.04763,0.242834539687906));
#7225=CARTESIAN_POINT('Ctrl Pts',(0.989696097314,-0.04763,-0.242834539687907));
#7226=CARTESIAN_POINT('Ctrl Pts',(0.990332542620729,-0.0609922781173483,
-0.24024064412003));
#7227=CARTESIAN_POINT('Ctrl Pts',(0.991238884025248,-0.0742967091364493,
-0.236509675094874));
#7228=CARTESIAN_POINT('Ctrl Pts',(0.994830026707808,-0.115492077056649,
-0.221129100087819));
#7229=CARTESIAN_POINT('Ctrl Pts',(0.998375294985966,-0.141695629206859,
-0.205111543747588));
#7230=CARTESIAN_POINT('Ctrl Pts',(1.00492400591205,-0.181890537957859,-0.169940289819232));
#7231=CARTESIAN_POINT('Ctrl Pts',(1.00869718865384,-0.201072148666545,-0.1465689792446));
#7232=CARTESIAN_POINT('Ctrl Pts',(1.01358704779679,-0.223955109275652,-0.106909345252087));
#7233=CARTESIAN_POINT('Ctrl Pts',(1.0156297872271,-0.232742381310829,-0.0861971848975942));
#7234=CARTESIAN_POINT('Ctrl Pts',(1.01837060663223,-0.244234834628584,-0.0430711894098823));
#7235=CARTESIAN_POINT('Ctrl Pts',(1.019052,-0.246942143572133,-0.0206568624125607));
#7236=CARTESIAN_POINT('Ctrl Pts',(1.019052,-0.246942143572133,0.0206568624125607));
#7237=CARTESIAN_POINT('Ctrl Pts',(1.01837060663223,-0.244234834628584,0.0430711894098823));
#7238=CARTESIAN_POINT('Ctrl Pts',(1.0156297872271,-0.232742381310829,0.0861971848975942));
#7239=CARTESIAN_POINT('Ctrl Pts',(1.01358704779679,-0.223955109275652,0.106909345252087));
#7240=CARTESIAN_POINT('Ctrl Pts',(1.00869718865384,-0.201072148666545,0.1465689792446));
#7241=CARTESIAN_POINT('Ctrl Pts',(1.00492400591205,-0.181890537957859,0.169940289819232));
#7242=CARTESIAN_POINT('Ctrl Pts',(0.998375294985966,-0.141695629206859,
0.205111543747588));
#7243=CARTESIAN_POINT('Ctrl Pts',(0.994830026707808,-0.115492077056649,
0.221129100087819));
#7244=CARTESIAN_POINT('Ctrl Pts',(0.991238884025248,-0.0742967091364492,
0.236509675094874));
#7245=CARTESIAN_POINT('Ctrl Pts',(0.990332542620729,-0.0609922781173483,
0.24024064412003));
#7246=CARTESIAN_POINT('Ctrl Pts',(0.989696097314,-0.04763,0.242834539687907));
#7247=CARTESIAN_POINT('Origin',(0.,-0.04763,0.));
#7248=CARTESIAN_POINT('Origin',(0.,-0.04763,0.));
#7249=CARTESIAN_POINT('',(0.238183666596899,-0.04763,0.951592097314));
#7250=CARTESIAN_POINT('Origin',(0.,-0.04763,0.));
#7251=CARTESIAN_POINT('Origin',(-1.94289029309402E-16,-0.04763,1.));
#7252=CARTESIAN_POINT('Origin',(-1.94289029309402E-16,0.,1.));
#7253=CARTESIAN_POINT('',(-0.2381836665969,-0.04763,0.951592097314));
#7254=CARTESIAN_POINT('Ctrl Pts',(-0.238183666596899,-0.0476299999999999,
0.951592097314));
#7255=CARTESIAN_POINT('Ctrl Pts',(-0.233157223576062,-0.0740444353928835,
0.952850216871763));
#7256=CARTESIAN_POINT('Ctrl Pts',(-0.223801617934946,-0.0999305678883309,
0.955173119738174));
#7257=CARTESIAN_POINT('Ctrl Pts',(-0.199966927975188,-0.142345102874864,
0.960411259488514));
#7258=CARTESIAN_POINT('Ctrl Pts',(-0.1868781821531,-0.159766064500479,0.963103647174702));
#7259=CARTESIAN_POINT('Ctrl Pts',(-0.15681442133453,-0.190326085855194,
0.968453058988463));
#7260=CARTESIAN_POINT('Ctrl Pts',(-0.139836317888043,-0.203463743702801,
0.971100730005489));
#7261=CARTESIAN_POINT('Ctrl Pts',(-0.104422493053067,-0.224161999508995,
0.975530745318961));
#7262=CARTESIAN_POINT('Ctrl Pts',(-0.0842175114474176,-0.232861760990032,
0.977553872336861));
#7263=CARTESIAN_POINT('Ctrl Pts',(-0.0421062857595701,-0.244251601209411,
0.980270995488453));
#7264=CARTESIAN_POINT('Ctrl Pts',(-0.0201990724523197,-0.246942143572133,
0.980948));
#7265=CARTESIAN_POINT('Ctrl Pts',(0.020199072452319,-0.246942143572133,
0.980948));
#7266=CARTESIAN_POINT('Ctrl Pts',(0.0421062857595694,-0.244251601209411,
0.980270995488454));
#7267=CARTESIAN_POINT('Ctrl Pts',(0.0842175114474169,-0.232861760990032,
0.977553872336861));
#7268=CARTESIAN_POINT('Ctrl Pts',(0.104422493053067,-0.224161999508995,
0.975530745318961));
#7269=CARTESIAN_POINT('Ctrl Pts',(0.139836317888042,-0.203463743702801,
0.971100730005489));
#7270=CARTESIAN_POINT('Ctrl Pts',(0.15681442133453,-0.190326085855194,0.968453058988463));
#7271=CARTESIAN_POINT('Ctrl Pts',(0.1868781821531,-0.15976606450048,0.963103647174702));
#7272=CARTESIAN_POINT('Ctrl Pts',(0.199966927975188,-0.142345102874864,
0.960411259488514));
#7273=CARTESIAN_POINT('Ctrl Pts',(0.223801617934945,-0.0999305678883309,
0.955173119738174));
#7274=CARTESIAN_POINT('Ctrl Pts',(0.233157223576061,-0.0740444353928835,
0.952850216871763));
#7275=CARTESIAN_POINT('Ctrl Pts',(0.238183666596899,-0.0476299999999999,
0.951592097314));
#7276=CARTESIAN_POINT('Origin',(-1.94289029309402E-16,-0.04763,1.));
#7277=CARTESIAN_POINT('Origin',(0.,-0.04763,0.));
#7278=CARTESIAN_POINT('',(-0.504455939115715,-0.04763,0.841298510752802));
#7279=CARTESIAN_POINT('Origin',(0.,-0.04763,0.));
#7280=CARTESIAN_POINT('Origin',(-0.707106781186548,-0.04763,0.707106781186547));
#7281=CARTESIAN_POINT('Origin',(-0.707106781186548,0.,0.707106781186547));
#7282=CARTESIAN_POINT('',(-0.841298510752802,-0.04763,0.504455939115715));
#7283=CARTESIAN_POINT('Ctrl Pts',(-0.841298510752802,-0.04763,0.504455939115715));
#7284=CARTESIAN_POINT('Ctrl Pts',(-0.838633903678357,-0.0740444353928835,
0.508899795931835));
#7285=CARTESIAN_POINT('Ctrl Pts',(-0.833661031856294,-0.0999305678883309,
0.517157748491652));
#7286=CARTESIAN_POINT('Ctrl Pts',(-0.820511285096538,-0.142345102874864,
0.537715343527944));
#7287=CARTESIAN_POINT('Ctrl Pts',(-0.813159949759,-0.159766064500479,0.548874290046456));
#7288=CARTESIAN_POINT('Ctrl Pts',(-0.795684265985089,-0.190326085855194,
0.573915184558107));
#7289=CARTESIAN_POINT('Ctrl Pts',(-0.78555112003688,-0.203463743702801,
0.587792702767295));
#7290=CARTESIAN_POINT('Ctrl Pts',(-0.763642258217233,-0.224161999508995,
0.615966552324775));
#7291=CARTESIAN_POINT('Ctrl Pts',(-0.750785745543687,-0.232861760990032,
0.631684198665438));
#7292=CARTESIAN_POINT('Ctrl Pts',(-0.722929908501543,-0.244251601209411,
0.663382628119203));
#7293=CARTESIAN_POINT('Ctrl Pts',(-0.707917883896095,-0.246942143572133,
0.679352081686668));
#7294=CARTESIAN_POINT('Ctrl Pts',(-0.679352081686668,-0.246942143572133,
0.707917883896095));
#7295=CARTESIAN_POINT('Ctrl Pts',(-0.663382628119203,-0.244251601209411,
0.722929908501544));
#7296=CARTESIAN_POINT('Ctrl Pts',(-0.631684198665438,-0.232861760990031,
0.750785745543687));
#7297=CARTESIAN_POINT('Ctrl Pts',(-0.615966552324775,-0.224161999508995,
0.763642258217233));
#7298=CARTESIAN_POINT('Ctrl Pts',(-0.587792702767295,-0.203463743702801,
0.78555112003688));
#7299=CARTESIAN_POINT('Ctrl Pts',(-0.573915184558107,-0.190326085855194,
0.795684265985088));
#7300=CARTESIAN_POINT('Ctrl Pts',(-0.548874290046456,-0.159766064500479,
0.813159949759));
#7301=CARTESIAN_POINT('Ctrl Pts',(-0.537715343527944,-0.142345102874864,
0.820511285096538));
#7302=CARTESIAN_POINT('Ctrl Pts',(-0.517157748491652,-0.0999305678883309,
0.833661031856294));
#7303=CARTESIAN_POINT('Ctrl Pts',(-0.508899795931835,-0.0740444353928835,
0.838633903678357));
#7304=CARTESIAN_POINT('Ctrl Pts',(-0.504455939115716,-0.04763,0.841298510752801));
#7305=CARTESIAN_POINT('Origin',(-0.707106781186548,-0.04763,0.707106781186547));
#7306=CARTESIAN_POINT('Origin',(0.,-0.04763,0.));
#7307=CARTESIAN_POINT('',(-0.951592097314,-0.04763,0.238183666596899));
#7308=CARTESIAN_POINT('Origin',(0.,-0.04763,0.));
#7309=CARTESIAN_POINT('Origin',(-1.,-0.04763,-1.11022302462516E-16));
#7310=CARTESIAN_POINT('Origin',(-1.,0.,-1.11022302462516E-16));
#7311=CARTESIAN_POINT('',(-0.951592097314,-0.04763,-0.2381836665969));
#7312=CARTESIAN_POINT('',(-0.980948,-0.246942143572133,1.08514323328844E-18));
#7313=CARTESIAN_POINT('Ctrl Pts',(-0.951592097314,-0.04763,-0.238183666596899));
#7314=CARTESIAN_POINT('Ctrl Pts',(-0.952850216871763,-0.0740444353928835,
-0.233157223576062));
#7315=CARTESIAN_POINT('Ctrl Pts',(-0.955173119738174,-0.0999305678883309,
-0.223801617934946));
#7316=CARTESIAN_POINT('Ctrl Pts',(-0.960411259488514,-0.142345102874864,
-0.199966927975188));
#7317=CARTESIAN_POINT('Ctrl Pts',(-0.963103647174702,-0.159766064500479,
-0.1868781821531));
#7318=CARTESIAN_POINT('Ctrl Pts',(-0.968453058988463,-0.190326085855194,
-0.15681442133453));
#7319=CARTESIAN_POINT('Ctrl Pts',(-0.971100730005489,-0.203463743702801,
-0.139836317888043));
#7320=CARTESIAN_POINT('Ctrl Pts',(-0.975530745318961,-0.224161999508995,
-0.104422493053067));
#7321=CARTESIAN_POINT('Ctrl Pts',(-0.977553872336861,-0.232861760990032,
-0.0842175114474175));
#7322=CARTESIAN_POINT('Ctrl Pts',(-0.980270995488453,-0.244251601209411,
-0.0421062857595699));
#7323=CARTESIAN_POINT('Ctrl Pts',(-0.980948,-0.246942143572133,-0.0201990724523195));
#7324=CARTESIAN_POINT('Ctrl Pts',(-0.980948,-0.246942143572133,-1.17961196366423E-16));
#7325=CARTESIAN_POINT('Origin',(-1.,-0.04763,-1.11022302462516E-16));
#7326=CARTESIAN_POINT('Ctrl Pts',(-0.980948,-0.246942143572133,-1.17961196366423E-16));
#7327=CARTESIAN_POINT('Ctrl Pts',(-0.980948,-0.246942143572133,0.0201990724523192));
#7328=CARTESIAN_POINT('Ctrl Pts',(-0.980270995488453,-0.244251601209411,
0.0421062857595695));
#7329=CARTESIAN_POINT('Ctrl Pts',(-0.977553872336861,-0.232861760990032,
0.0842175114474169));
#7330=CARTESIAN_POINT('Ctrl Pts',(-0.975530745318961,-0.224161999508995,
0.104422493053066));
#7331=CARTESIAN_POINT('Ctrl Pts',(-0.971100730005489,-0.203463743702801,
0.139836317888042));
#7332=CARTESIAN_POINT('Ctrl Pts',(-0.968453058988463,-0.190326085855194,
0.15681442133453));
#7333=CARTESIAN_POINT('Ctrl Pts',(-0.963103647174702,-0.15976606450048,
0.1868781821531));
#7334=CARTESIAN_POINT('Ctrl Pts',(-0.960411259488514,-0.142345102874864,
0.199966927975188));
#7335=CARTESIAN_POINT('Ctrl Pts',(-0.955173119738174,-0.099930567888331,
0.223801617934945));
#7336=CARTESIAN_POINT('Ctrl Pts',(-0.952850216871763,-0.0740444353928835,
0.233157223576061));
#7337=CARTESIAN_POINT('Ctrl Pts',(-0.951592097314,-0.04763,0.238183666596899));
#7338=CARTESIAN_POINT('Origin',(0.,-0.04763,0.));
#7339=CARTESIAN_POINT('',(-0.841298510752802,-0.04763,-0.504455939115715));
#7340=CARTESIAN_POINT('Origin',(0.,-0.04763,0.));
#7341=CARTESIAN_POINT('Origin',(-0.707106781186547,-0.04763,-0.707106781186548));
#7342=CARTESIAN_POINT('Origin',(-0.707106781186547,0.,-0.707106781186548));
#7343=CARTESIAN_POINT('',(-0.504455939115715,-0.04763,-0.841298510752802));
#7344=CARTESIAN_POINT('Ctrl Pts',(-0.504455939115715,-0.04763,-0.841298510752802));
#7345=CARTESIAN_POINT('Ctrl Pts',(-0.508899795931835,-0.0740444353928835,
-0.838633903678357));
#7346=CARTESIAN_POINT('Ctrl Pts',(-0.517157748491652,-0.0999305678883309,
-0.833661031856294));
#7347=CARTESIAN_POINT('Ctrl Pts',(-0.537715343527944,-0.142345102874864,
-0.820511285096538));
#7348=CARTESIAN_POINT('Ctrl Pts',(-0.548874290046456,-0.159766064500479,
-0.813159949759));
#7349=CARTESIAN_POINT('Ctrl Pts',(-0.573915184558107,-0.190326085855194,
-0.795684265985089));
#7350=CARTESIAN_POINT('Ctrl Pts',(-0.587792702767295,-0.203463743702801,
-0.78555112003688));
#7351=CARTESIAN_POINT('Ctrl Pts',(-0.615966552324775,-0.224161999508995,
-0.763642258217233));
#7352=CARTESIAN_POINT('Ctrl Pts',(-0.631684198665438,-0.232861760990032,
-0.750785745543687));
#7353=CARTESIAN_POINT('Ctrl Pts',(-0.663382628119203,-0.244251601209411,
-0.722929908501543));
#7354=CARTESIAN_POINT('Ctrl Pts',(-0.679352081686668,-0.246942143572133,
-0.707917883896095));
#7355=CARTESIAN_POINT('Ctrl Pts',(-0.707917883896095,-0.246942143572133,
-0.679352081686668));
#7356=CARTESIAN_POINT('Ctrl Pts',(-0.722929908501543,-0.244251601209411,
-0.663382628119203));
#7357=CARTESIAN_POINT('Ctrl Pts',(-0.750785745543687,-0.232861760990032,
-0.631684198665439));
#7358=CARTESIAN_POINT('Ctrl Pts',(-0.763642258217232,-0.224161999508995,
-0.615966552324775));
#7359=CARTESIAN_POINT('Ctrl Pts',(-0.78555112003688,-0.203463743702801,
-0.587792702767295));
#7360=CARTESIAN_POINT('Ctrl Pts',(-0.795684265985088,-0.190326085855194,
-0.573915184558107));
#7361=CARTESIAN_POINT('Ctrl Pts',(-0.813159949759,-0.15976606450048,-0.548874290046456));
#7362=CARTESIAN_POINT('Ctrl Pts',(-0.820511285096538,-0.142345102874864,
-0.537715343527944));
#7363=CARTESIAN_POINT('Ctrl Pts',(-0.833661031856294,-0.0999305678883311,
-0.517157748491652));
#7364=CARTESIAN_POINT('Ctrl Pts',(-0.838633903678357,-0.0740444353928836,
-0.508899795931835));
#7365=CARTESIAN_POINT('Ctrl Pts',(-0.841298510752801,-0.04763,-0.504455939115715));
#7366=CARTESIAN_POINT('Origin',(-0.707106781186547,-0.04763,-0.707106781186548));
#7367=CARTESIAN_POINT('Origin',(0.,-0.04763,0.));
#7368=CARTESIAN_POINT('',(-0.238183666596899,-0.04763,-0.951592097314));
#7369=CARTESIAN_POINT('Origin',(0.,-0.04763,0.));
#7370=CARTESIAN_POINT('Origin',(5.55111512312578E-17,-0.04763,-1.));
#7371=CARTESIAN_POINT('Origin',(5.55111512312578E-17,0.,-1.));
#7372=CARTESIAN_POINT('',(0.238183666596899,-0.04763,-0.951592097314));
#7373=CARTESIAN_POINT('Ctrl Pts',(0.238183666596899,-0.04763,-0.951592097314));
#7374=CARTESIAN_POINT('Ctrl Pts',(0.233157223576062,-0.0740444353928835,
-0.952850216871763));
#7375=CARTESIAN_POINT('Ctrl Pts',(0.223801617934946,-0.099930567888331,
-0.955173119738174));
#7376=CARTESIAN_POINT('Ctrl Pts',(0.199966927975188,-0.142345102874864,
-0.960411259488514));
#7377=CARTESIAN_POINT('Ctrl Pts',(0.1868781821531,-0.15976606450048,-0.963103647174702));
#7378=CARTESIAN_POINT('Ctrl Pts',(0.15681442133453,-0.190326085855194,-0.968453058988463));
#7379=CARTESIAN_POINT('Ctrl Pts',(0.139836317888042,-0.203463743702801,
-0.971100730005489));
#7380=CARTESIAN_POINT('Ctrl Pts',(0.104422493053067,-0.224161999508995,
-0.975530745318961));
#7381=CARTESIAN_POINT('Ctrl Pts',(0.0842175114474173,-0.232861760990032,
-0.977553872336861));
#7382=CARTESIAN_POINT('Ctrl Pts',(0.0421062857595698,-0.244251601209411,
-0.980270995488453));
#7383=CARTESIAN_POINT('Ctrl Pts',(0.0201990724523194,-0.246942143572133,
-0.980948));
#7384=CARTESIAN_POINT('Ctrl Pts',(-0.0201990724523193,-0.246942143572133,
-0.980948));
#7385=CARTESIAN_POINT('Ctrl Pts',(-0.0421062857595697,-0.244251601209411,
-0.980270995488453));
#7386=CARTESIAN_POINT('Ctrl Pts',(-0.0842175114474171,-0.232861760990032,
-0.977553872336861));
#7387=CARTESIAN_POINT('Ctrl Pts',(-0.104422493053067,-0.224161999508995,
-0.975530745318961));
#7388=CARTESIAN_POINT('Ctrl Pts',(-0.139836317888042,-0.203463743702801,
-0.971100730005489));
#7389=CARTESIAN_POINT('Ctrl Pts',(-0.15681442133453,-0.190326085855194,
-0.968453058988463));
#7390=CARTESIAN_POINT('Ctrl Pts',(-0.1868781821531,-0.15976606450048,-0.963103647174702));
#7391=CARTESIAN_POINT('Ctrl Pts',(-0.199966927975188,-0.142345102874864,
-0.960411259488514));
#7392=CARTESIAN_POINT('Ctrl Pts',(-0.223801617934945,-0.099930567888331,
-0.955173119738174));
#7393=CARTESIAN_POINT('Ctrl Pts',(-0.233157223576062,-0.0740444353928835,
-0.952850216871763));
#7394=CARTESIAN_POINT('Ctrl Pts',(-0.238183666596899,-0.0476299999999999,
-0.951592097314));
#7395=CARTESIAN_POINT('Origin',(5.55111512312578E-17,-0.04763,-1.));
#7396=CARTESIAN_POINT('Origin',(0.,-0.04763,0.));
#7397=CARTESIAN_POINT('',(0.504455939115715,-0.04763,-0.841298510752802));
#7398=CARTESIAN_POINT('Origin',(0.,-0.04763,0.));
#7399=CARTESIAN_POINT('Origin',(0.707106781186548,-0.04763,-0.707106781186547));
#7400=CARTESIAN_POINT('Origin',(0.707106781186548,0.,-0.707106781186547));
#7401=CARTESIAN_POINT('',(0.841298510752802,-0.04763,-0.504455939115715));
#7402=CARTESIAN_POINT('Ctrl Pts',(0.841298510752802,-0.04763,-0.504455939115715));
#7403=CARTESIAN_POINT('Ctrl Pts',(0.838633903678357,-0.0740444353928835,
-0.508899795931835));
#7404=CARTESIAN_POINT('Ctrl Pts',(0.833661031856294,-0.0999305678883309,
-0.517157748491652));
#7405=CARTESIAN_POINT('Ctrl Pts',(0.820511285096538,-0.142345102874864,
-0.537715343527944));
#7406=CARTESIAN_POINT('Ctrl Pts',(0.813159949759,-0.159766064500479,-0.548874290046456));
#7407=CARTESIAN_POINT('Ctrl Pts',(0.795684265985088,-0.190326085855194,
-0.573915184558107));
#7408=CARTESIAN_POINT('Ctrl Pts',(0.78555112003688,-0.203463743702801,-0.587792702767295));
#7409=CARTESIAN_POINT('Ctrl Pts',(0.763642258217233,-0.224161999508995,
-0.615966552324775));
#7410=CARTESIAN_POINT('Ctrl Pts',(0.750785745543687,-0.232861760990032,
-0.631684198665438));
#7411=CARTESIAN_POINT('Ctrl Pts',(0.722929908501543,-0.244251601209411,
-0.663382628119203));
#7412=CARTESIAN_POINT('Ctrl Pts',(0.707917883896095,-0.246942143572133,
-0.679352081686668));
#7413=CARTESIAN_POINT('Ctrl Pts',(0.679352081686668,-0.246942143572133,
-0.707917883896095));
#7414=CARTESIAN_POINT('Ctrl Pts',(0.663382628119203,-0.244251601209411,
-0.722929908501543));
#7415=CARTESIAN_POINT('Ctrl Pts',(0.631684198665438,-0.232861760990032,
-0.750785745543687));
#7416=CARTESIAN_POINT('Ctrl Pts',(0.615966552324775,-0.224161999508995,
-0.763642258217232));
#7417=CARTESIAN_POINT('Ctrl Pts',(0.587792702767295,-0.203463743702801,
-0.78555112003688));
#7418=CARTESIAN_POINT('Ctrl Pts',(0.573915184558107,-0.190326085855194,
-0.795684265985088));
#7419=CARTESIAN_POINT('Ctrl Pts',(0.548874290046456,-0.159766064500479,
-0.813159949759));
#7420=CARTESIAN_POINT('Ctrl Pts',(0.537715343527944,-0.142345102874864,
-0.820511285096538));
#7421=CARTESIAN_POINT('Ctrl Pts',(0.517157748491652,-0.099930567888331,
-0.833661031856294));
#7422=CARTESIAN_POINT('Ctrl Pts',(0.508899795931835,-0.0740444353928835,
-0.838633903678357));
#7423=CARTESIAN_POINT('Ctrl Pts',(0.504455939115715,-0.04763,-0.841298510752801));
#7424=CARTESIAN_POINT('Origin',(0.707106781186548,-0.04763,-0.707106781186547));
#7425=CARTESIAN_POINT('Origin',(0.,-0.166705,0.));
#7426=CARTESIAN_POINT('',(-0.980948,-0.28578,1.20131482833E-16));
#7427=CARTESIAN_POINT('Origin',(0.,-0.28578,0.));
#7428=CARTESIAN_POINT('',(-0.980948,-0.166705,1.20131482833E-16));
#7429=CARTESIAN_POINT('',(0.951592097314,-0.04763,0.238183666596899));
#7430=CARTESIAN_POINT('Origin',(0.,-0.04763,0.));
#7431=CARTESIAN_POINT('',(0.951592097314,-0.04763,-0.238183666596899));
#7432=CARTESIAN_POINT('Ctrl Pts',(0.951592097314,-0.04763,0.238183666596899));
#7433=CARTESIAN_POINT('Ctrl Pts',(0.952850216871763,-0.0740444353928835,
0.233157223576062));
#7434=CARTESIAN_POINT('Ctrl Pts',(0.955173119738174,-0.099930567888331,
0.223801617934945));
#7435=CARTESIAN_POINT('Ctrl Pts',(0.960411259488514,-0.142345102874864,
0.199966927975188));
#7436=CARTESIAN_POINT('Ctrl Pts',(0.963103647174702,-0.15976606450048,0.1868781821531));
#7437=CARTESIAN_POINT('Ctrl Pts',(0.968453058988463,-0.190326085855194,
0.15681442133453));
#7438=CARTESIAN_POINT('Ctrl Pts',(0.971100730005489,-0.203463743702801,
0.139836317888042));
#7439=CARTESIAN_POINT('Ctrl Pts',(0.975530745318961,-0.224161999508995,
0.104422493053067));
#7440=CARTESIAN_POINT('Ctrl Pts',(0.977553872336861,-0.232861760990032,
0.0842175114474172));
#7441=CARTESIAN_POINT('Ctrl Pts',(0.980270995488453,-0.244251601209411,
0.0421062857595697));
#7442=CARTESIAN_POINT('Ctrl Pts',(0.980948,-0.246942143572133,0.0201990724523194));
#7443=CARTESIAN_POINT('Ctrl Pts',(0.980948,-0.246942143572133,-0.0201990724523194));
#7444=CARTESIAN_POINT('Ctrl Pts',(0.980270995488453,-0.244251601209411,
-0.0421062857595697));
#7445=CARTESIAN_POINT('Ctrl Pts',(0.977553872336861,-0.232861760990032,
-0.0842175114474172));
#7446=CARTESIAN_POINT('Ctrl Pts',(0.975530745318961,-0.224161999508995,
-0.104422493053067));
#7447=CARTESIAN_POINT('Ctrl Pts',(0.971100730005489,-0.203463743702801,
-0.139836317888042));
#7448=CARTESIAN_POINT('Ctrl Pts',(0.968453058988463,-0.190326085855194,
-0.15681442133453));
#7449=CARTESIAN_POINT('Ctrl Pts',(0.963103647174702,-0.15976606450048,-0.1868781821531));
#7450=CARTESIAN_POINT('Ctrl Pts',(0.960411259488514,-0.142345102874864,
-0.199966927975188));
#7451=CARTESIAN_POINT('Ctrl Pts',(0.955173119738174,-0.099930567888331,
-0.223801617934945));
#7452=CARTESIAN_POINT('Ctrl Pts',(0.952850216871763,-0.0740444353928835,
-0.233157223576062));
#7453=CARTESIAN_POINT('Ctrl Pts',(0.951592097314,-0.0476299999999999,-0.238183666596899));
#7454=CARTESIAN_POINT('Origin',(0.,-0.04763,0.));
#7455=CARTESIAN_POINT('Origin',(0.,-0.04763,0.));
#7456=CARTESIAN_POINT('Origin',(1.,-0.04763,0.));
#7457=CARTESIAN_POINT('Origin',(1.,0.,0.));
#7458=CARTESIAN_POINT('Origin',(1.,-0.04763,0.));
#7459=CARTESIAN_POINT('Origin',(0.,-0.28578,0.));
#7460=CARTESIAN_POINT('Origin',(0.,-0.04763,0.));
#7772=UNCERTAINTY_MEASURE_WITH_UNIT(LENGTH_MEASURE(0.001),#7807,
'DISTANCE_ACCURACY_VALUE',
'Maximum model space distance between geometric entities at asserted c
onnectivities');
#7782=UNCERTAINTY_MEASURE_WITH_UNIT(LENGTH_MEASURE(0.001),#7807,
'DISTANCE_ACCURACY_VALUE',
'Maximum model space distance between geometric entities at asserted c
onnectivities');
#7796=(
GEOMETRIC_REPRESENTATION_CONTEXT(3)
GLOBAL_UNCERTAINTY_ASSIGNED_CONTEXT((#7772))
GLOBAL_UNIT_ASSIGNED_CONTEXT((#7807,#7809,#7810))
REPRESENTATION_CONTEXT('','3D')
);
#7806=(
GEOMETRIC_REPRESENTATION_CONTEXT(3)
GLOBAL_UNCERTAINTY_ASSIGNED_CONTEXT((#7782))
GLOBAL_UNIT_ASSIGNED_CONTEXT((#7807,#7809,#7810))
REPRESENTATION_CONTEXT('','3D')
);
#7807=(
LENGTH_UNIT()
NAMED_UNIT(*)
SI_UNIT(.CENTI.,.METRE.)
);
#7809=(
NAMED_UNIT(*)
PLANE_ANGLE_UNIT()
SI_UNIT($,.RADIAN.)
);
#7810=(
NAMED_UNIT(*)
SI_UNIT($,.STERADIAN.)
SOLID_ANGLE_UNIT()
);
#7824=SHAPE_DEFINITION_REPRESENTATION(#7847,#7923);
#7847=PRODUCT_DEFINITION_SHAPE('',$,#7947);
#7923=SHAPE_REPRESENTATION('',(#4676),#7796);
#7933=PRODUCT_DEFINITION_CONTEXT('part definition',#8004,'design');
#7947=PRODUCT_DEFINITION('Cage','Cage',#7970,#7933);
#7970=PRODUCT_DEFINITION_FORMATION('',$,#8019);
#8004=APPLICATION_CONTEXT(
'Core Data for Automotive Mechanical Design Process');
#8005=PRODUCT_CONTEXT('part definition',#8004,'mechanical');
#8019=PRODUCT('Cage','Cage','Cage',(#8005));
#8085=COLOUR_RGB('Grey',0.48,0.52,0.57);
#8086=FILL_AREA_STYLE_COLOUR('',#8085);
#8087=FILL_AREA_STYLE('',(#8086));
#8088=SURFACE_STYLE_FILL_AREA(#8087);
#8089=SURFACE_SIDE_STYLE('',(#8088));
#8090=SURFACE_STYLE_USAGE(.BOTH.,#8089);
#8091=PRESENTATION_STYLE_ASSIGNMENT((#8090));
ENDSEC;
END-ISO-10303-21;
